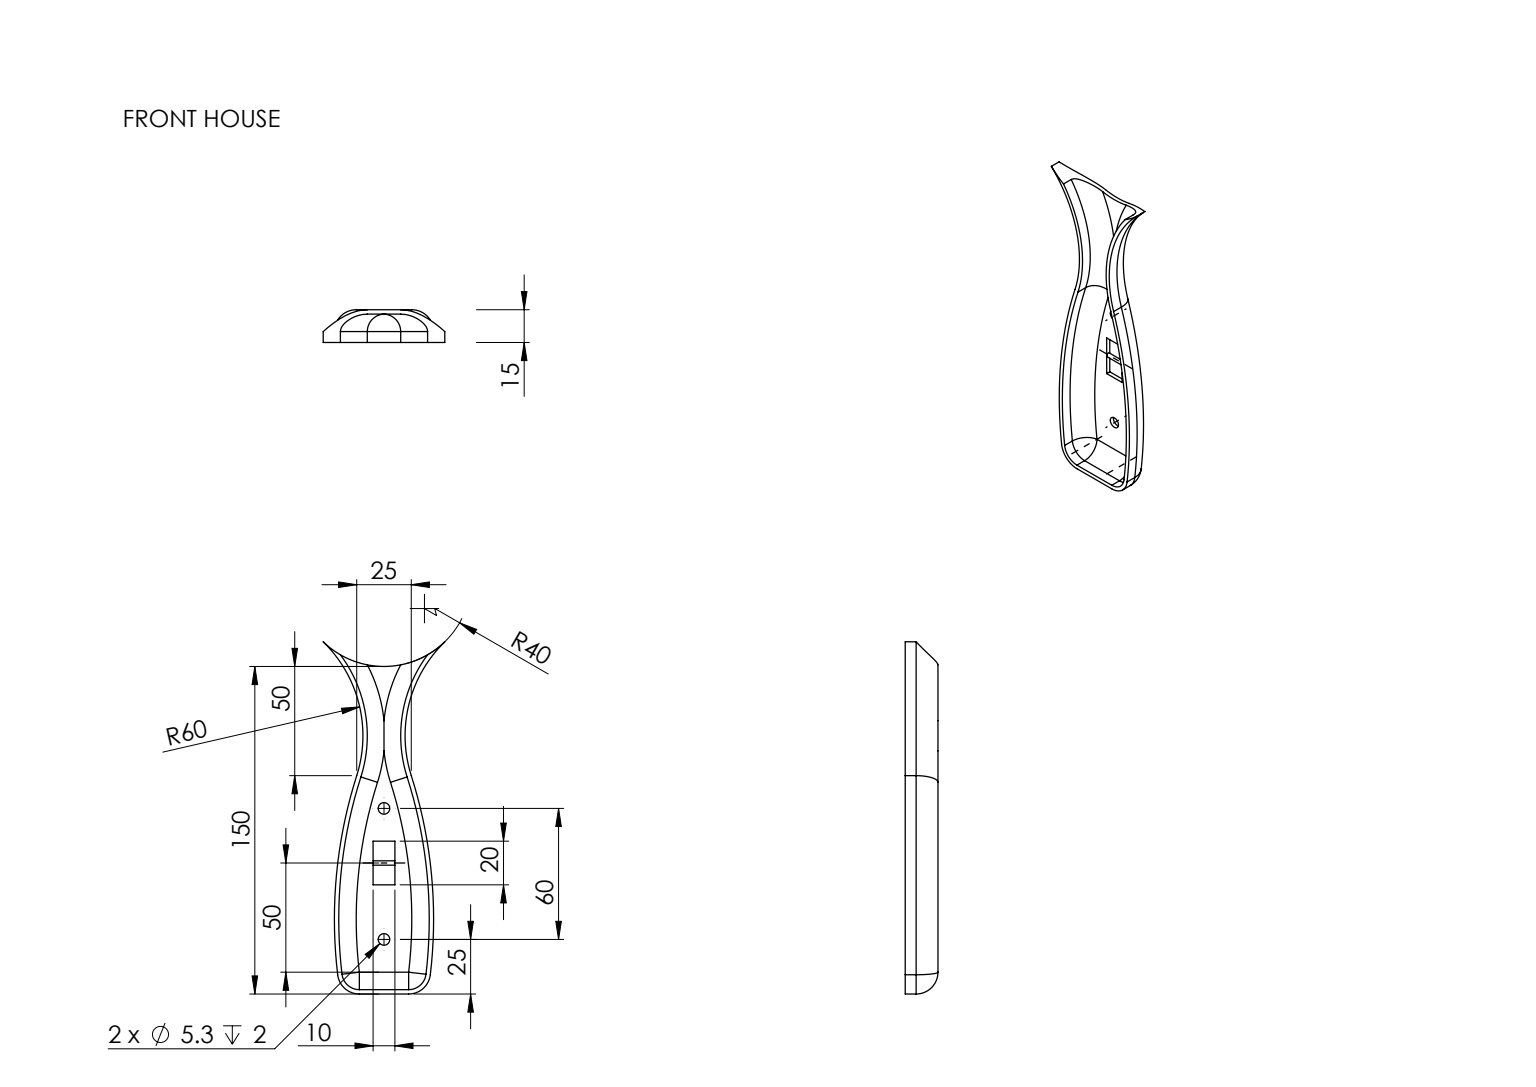
ISO-10303-21;
HEADER;
FILE_DESCRIPTION (('STEP AP214'),
    '1' );
FILE_NAME ('front house.step',
    '2026-10-04T13:31:42',
    ( '' ),
    ( '' ),
    'SwSTEP 2.0',
    'SolidWorks 2026',
    '' );
FILE_SCHEMA (( 'AUTOMOTIVE_DESIGN' ));
ENDSEC;

DATA;
#31=DIRECTION ( 'NONE',  ( 0.000000000000000000, 0.000000000000000000, 1.000000000000000000 ) ) ;
#221=EDGE_CURVE ( 'NONE', #165210, #193478, #178958, .T. ) ;
#227=CARTESIAN_POINT ( 'NONE',  ( 69.65682714487590488, -71.74905178543389184, -4.999999999999999112 ) ) ;
#394=ADVANCED_FACE ( 'NONE', ( #34064 ), #127044, .F. ) ;
#780=DIRECTION ( 'NONE',  ( 0.000000000000000000, 0.000000000000000000, 1.000000000000000000 ) ) ;
#955=EDGE_CURVE ( 'NONE', #12036, #40598, #167128, .T. ) ;
#999=ORIENTED_EDGE ( 'NONE', *, *, #31053, .F. ) ;
#1017=VECTOR ( 'NONE', #142739, 1000.000000000000000 ) ;
#1085=CARTESIAN_POINT ( 'NONE',  ( 2.973862142520697471, -93.04182470242777470, -4.999999999999999112 ) ) ;
#1208=CARTESIAN_POINT ( 'NONE',  ( -193.3062444957834884, -155.7167183371838064, -4.999999999999999112 ) ) ;
#1246=DIRECTION ( 'NONE',  ( 0.000000000000000000, 0.000000000000000000, -1.000000000000000000 ) ) ;
#1328=( LENGTH_UNIT ( ) NAMED_UNIT ( * ) SI_UNIT ( .MILLI., .METRE. ) );
#1396=AXIS2_PLACEMENT_3D ( 'NONE', #152271, #151292, #11796 ) ;
#1425=AXIS2_PLACEMENT_3D ( 'NONE', #179920, #53542, #83864 ) ;
#1725=ORIENTED_EDGE ( 'NONE', *, *, #84050, .T. ) ;
#1873=CARTESIAN_POINT ( 'NONE',  ( 18.50421606877890923, -35.46346162465770391, -8.316515678940758605 ) ) ;
#2039=ORIENTED_EDGE ( 'NONE', *, *, #94568, .T. ) ;
#2326=AXIS2_PLACEMENT_3D ( 'NONE', #102933, #86762, #132273 ) ;
#2374=CARTESIAN_POINT ( 'NONE',  ( 21.23184647844206197, -181.1785498424364675, 0.000000000000000000 ) ) ;
#2569=AXIS2_PLACEMENT_3D ( 'NONE', #195043, #118200, #101008 ) ;
#2600=CIRCLE ( 'NONE', #60618, 214.0437394197456342 ) ;
#3186=CARTESIAN_POINT ( 'NONE',  ( -4.999999999999999112, -140.0000000000000000, -15.00000000000000000 ) ) ;
#3248=FACE_OUTER_BOUND ( 'NONE', #133845, .T. ) ;
#3260=EDGE_CURVE ( 'NONE', #40834, #66675, #157727, .T. ) ;
#3607=CARTESIAN_POINT ( 'NONE',  ( 22.30855676328228654, -33.25042073255080766, -9.512168350472055778 ) ) ;
#3770=DIRECTION ( 'NONE',  ( 0.000000000000000000, 0.000000000000000000, 1.000000000000000000 ) ) ;
#3944=ORIENTED_EDGE ( 'NONE', *, *, #32795, .T. ) ;
#3998=DIRECTION ( 'NONE',  ( -0.1178549842436482503, 0.9930308165857338887, -1.226674847570000151E-16 ) ) ;
#4010=( NAMED_UNIT ( * ) SI_UNIT ( $, .STERADIAN. ) SOLID_ANGLE_UNIT ( ) );
#4197=DIRECTION ( 'NONE',  ( -1.000000000000000000, 0.000000000000000000, 0.000000000000000000 ) ) ;
#4394=EDGE_LOOP ( 'NONE', ( #77649, #111972, #192802, #188802 ) ) ;
#4402=ORIENTED_EDGE ( 'NONE', *, *, #164677, .T. ) ;
#4433=CARTESIAN_POINT ( 'NONE',  ( -4.622231866529366047E-30, -105.0000000000000000, -15.00000000000000000 ) ) ;
#4442=CARTESIAN_POINT ( 'NONE',  ( -7.652493125962417153, -39.26116846143397510, -13.00000000000000000 ) ) ;
#4543=CARTESIAN_POINT ( 'NONE',  ( -69.65682714487590488, -71.74905178543390605, -15.00000000000000000 ) ) ;
#4625=EDGE_CURVE ( 'NONE', #192038, #188447, #191917, .T. ) ;
#4663=CARTESIAN_POINT ( 'NONE',  ( -4.999999999999999112, -140.0000000000000000, -15.00000000000000000 ) ) ;
#4730=CIRCLE ( 'NONE', #36937, 214.0437394197456911 ) ;
#4808=ADVANCED_FACE ( 'NONE', ( #75423 ), #167452, .T. ) ;
#4872=ORIENTED_EDGE ( 'NONE', *, *, #119692, .T. ) ;
#5076=DIRECTION ( 'NONE',  ( 1.000000000000000000, -5.392603844284257652E-33, 0.000000000000000000 ) ) ;
#5235=CARTESIAN_POINT ( 'NONE',  ( 5.000000000000001776, -120.0000000000000142, 0.0009999999999992653654 ) ) ;
#5261=EDGE_CURVE ( 'NONE', #139926, #193517, #14400, .T. ) ;
#5267=FACE_OUTER_BOUND ( 'NONE', #180808, .T. ) ;
#5354=CIRCLE ( 'NONE', #118409, 40.00000000000002132 ) ;
#5434=CARTESIAN_POINT ( 'NONE',  ( -4.718528363748727840E-30, -105.0000000000000000, -13.00000000000000000 ) ) ;
#5444=CARTESIAN_POINT ( 'NONE',  ( -10.96632750431057879, -38.47313893329367573, -12.60384275245237617 ) ) ;
#5846=CARTESIAN_POINT ( 'NONE',  ( 14.06517603784871007, -37.45098900586879154, -11.50478690063030562 ) ) ;
#6002=( NAMED_UNIT ( * ) PLANE_ANGLE_UNIT ( ) SI_UNIT ( $, .RADIAN. ) );
#6237=DIRECTION ( 'NONE',  ( -5.392603844284257652E-33, 1.000000000000000000, 0.000000000000000000 ) ) ;
#6266=CYLINDRICAL_SURFACE ( 'NONE', #130179, 59.99999999999998579 ) ;
#6267=ORIENTED_EDGE ( 'NONE', *, *, #21840, .T. ) ;
#6497=DIRECTION ( 'NONE',  ( -1.000000000000000000, -4.336808689942018352E-17, 3.574525976782710619E-31 ) ) ;
#6556=DIRECTION ( 'NONE',  ( 0.000000000000000000, 0.000000000000000000, -1.000000000000000000 ) ) ;
#6627=VERTEX_POINT ( 'NONE', #57076 ) ;
#6820=FACE_OUTER_BOUND ( 'NONE', #145721, .T. ) ;
#6959=CARTESIAN_POINT ( 'NONE',  ( -9.720620470091368759, -38.81506340700470048, -14.89813575833734305 ) ) ;
#7058=MANIFOLD_SOLID_BREP ( 'AdvancedHole1', #101418 ) ;
#7224=DIRECTION ( 'NONE',  ( 1.000000000000000000, 0.000000000000000000, 0.000000000000000000 ) ) ;
#7386=EDGE_LOOP ( 'NONE', ( #176353, #78348, #99493, #52023, #74607 ) ) ;
#7454=LINE ( 'NONE', #67143, #166615 ) ;
#8020=DIRECTION ( 'NONE',  ( -1.000000000000000000, -5.267352820763006950E-15, 0.000000000000000000 ) ) ;
#8023=AXIS2_PLACEMENT_3D ( 'NONE', #149445, #135288, #120095 ) ;
#8299=ADVANCED_FACE ( 'NONE', ( #6820 ), #108199, .F. ) ;
#8310=EDGE_CURVE ( 'NONE', #132987, #99125, #22008, .T. ) ;
#8317=EDGE_LOOP ( 'NONE', ( #155924, #169926 ) ) ;
#8368=CIRCLE ( 'NONE', #104487, 69.99999999999997158 ) ;
#8438=ORIENTED_EDGE ( 'NONE', *, *, #48191, .F. ) ;
#8454=DIRECTION ( 'NONE',  ( -1.000000000000000000, 0.000000000000000000, 0.000000000000000000 ) ) ;
#8593=VERTEX_POINT ( 'NONE', #115010 ) ;
#8666=ORIENTED_EDGE ( 'NONE', *, *, #178067, .T. ) ;
#9000=CARTESIAN_POINT ( 'NONE',  ( -0.3431728551240714742, -71.74905178543389184, -4.999999999999999112 ) ) ;
#9041=CARTESIAN_POINT ( 'NONE',  ( 193.3062444957835453, -155.7167183371837496, -4.999999999999999112 ) ) ;
#9199=ADVANCED_FACE ( 'NONE', ( #12843 ), #74509, .F. ) ;
#9471=CARTESIAN_POINT ( 'NONE',  ( -18.05685959898565685, -35.69332804049738428, -8.787752958456431784 ) ) ;
#9484=DIRECTION ( 'NONE',  ( -1.000000000000000000, 4.336808689942018352E-17, 0.000000000000000000 ) ) ;
#9541=CARTESIAN_POINT ( 'NONE',  ( 5.000000000000000888, -140.0000000000000000, 0.0009999999999992653654 ) ) ;
#9567=DIRECTION ( 'NONE',  ( 0.000000000000000000, 0.000000000000000000, -1.000000000000000000 ) ) ;
#9619=CARTESIAN_POINT ( 'NONE',  ( 11.73776690369117937, -38.24261239843917082, -14.51832217641615586 ) ) ;
#9693=CARTESIAN_POINT ( 'NONE',  ( 19.97888994334924107, -34.65319547504297759, 0.000000000000000000 ) ) ;
#9945=PLANE ( 'NONE',  #95324 ) ;
#10213=CARTESIAN_POINT ( 'NONE',  ( -7.656827144875921753, -71.74905178543390605, -15.00000000000000000 ) ) ;
#10237=ORIENTED_EDGE ( 'NONE', *, *, #127999, .T. ) ;
#10262=FACE_OUTER_BOUND ( 'NONE', #193309, .T. ) ;
#10449=CARTESIAN_POINT ( 'NONE',  ( 5.000000000000000888, -140.0000000000000000, -15.00000000000000000 ) ) ;
#10474=ORIENTED_EDGE ( 'NONE', *, *, #142789, .T. ) ;
#10483=DIRECTION ( 'NONE',  ( 0.000000000000000000, -1.000000000000000000, 0.000000000000000000 ) ) ;
#10575=ADVANCED_FACE ( 'NONE', ( #143863 ), #188902, .T. ) ;
#10632=AXIS2_PLACEMENT_3D ( 'NONE', #1085, #62761, #79930 ) ;
#10770=CIRCLE ( 'NONE', #191582, 69.99999999999997158 ) ;
#11242=EDGE_LOOP ( 'NONE', ( #101594, #137434, #105999, #91375 ) ) ;
#11284=TOROIDAL_SURFACE ( 'NONE', #156599, 69.99999999999998579, 10.00000000000000000 ) ;
#11382=AXIS2_PLACEMENT_3D ( 'NONE', #132278, #86767, #89760 ) ;
#11477=CARTESIAN_POINT ( 'NONE',  ( -18.72120804366350555, -35.34920564451201841, -8.063943084929409366 ) ) ;
#11550=AXIS2_PLACEMENT_3D ( 'NONE', #60720, #15228, #76887 ) ;
#11796=DIRECTION ( 'NONE',  ( -1.000000000000000000, 5.392603844284257652E-33, 0.000000000000000000 ) ) ;
#11861=CARTESIAN_POINT ( 'NONE',  ( 5.000000000000000888, -140.0000000000000000, 0.0009999999999992653654 ) ) ;
#11911=CIRCLE ( 'NONE', #95864, 216.0437394197456911 ) ;
#11953=FACE_OUTER_BOUND ( 'NONE', #124538, .T. ) ;
#12010=PLANE ( 'NONE',  #96796 ) ;
#12035=CARTESIAN_POINT ( 'NONE',  ( 21.23184647844207618, -181.1785498424364675, -4.999999999999999112 ) ) ;
#12036=VERTEX_POINT ( 'NONE', #40450 ) ;
#12455=CIRCLE ( 'NONE', #177115, 216.0437394197456911 ) ;
#12473=CARTESIAN_POINT ( 'NONE',  ( -15.76296483128273707, -36.76812510865116934, -10.58138071059118701 ) ) ;
#12478=ORIENTED_EDGE ( 'NONE', *, *, #22446, .F. ) ;
#12843=FACE_OUTER_BOUND ( 'NONE', #7386, .T. ) ;
#12933=CARTESIAN_POINT ( 'NONE',  ( -3.573655867281984216E-15, 2.428612866367529932E-14, -13.00000000000000000 ) ) ;
#12963=DIRECTION ( 'NONE',  ( -1.000000000000000000, 0.000000000000000000, 0.000000000000000000 ) ) ;
#13167=ORIENTED_EDGE ( 'NONE', *, *, #59429, .F. ) ;
#13706=ADVANCED_FACE ( 'NONE', ( #135627 ), #151779, .T. ) ;
#13755=DIRECTION ( 'NONE',  ( -5.392603844284257652E-33, -1.000000000000000000, -0.000000000000000000 ) ) ;
#13813=ORIENTED_EDGE ( 'NONE', *, *, #31053, .T. ) ;
#13989=ORIENTED_EDGE ( 'NONE', *, *, #42025, .F. ) ;
#13996=EDGE_LOOP ( 'NONE', ( #152884, #135844, #78840, #26414, #124117, #87089 ) ) ;
#14043=ORIENTED_EDGE ( 'NONE', *, *, #118990, .F. ) ;
#14248=LINE ( 'NONE', #45591, #191110 ) ;
#14299=CARTESIAN_POINT ( 'NONE',  ( 5.000000000000001776, -130.0000000000000000, -15.00000000000000000 ) ) ;
#14379=ORIENTED_EDGE ( 'NONE', *, *, #143946, .T. ) ;
#14400=CIRCLE ( 'NONE', #49903, 1.000000000000000888 ) ;
#14416=FACE_OUTER_BOUND ( 'NONE', #72162, .T. ) ;
#14442=DIRECTION ( 'NONE',  ( 0.000000000000000000, 0.000000000000000000, 1.000000000000000000 ) ) ;
#14496=VERTEX_POINT ( 'NONE', #24871 ) ;
#14587=PRODUCT ( 'front house', 'front house', '', ( #99773 ) ) ;
#14624=EDGE_LOOP ( 'NONE', ( #60138, #151275, #103948, #169903 ) ) ;
#14670=ORIENTED_EDGE ( 'NONE', *, *, #30090, .T. ) ;
#15059=DIRECTION ( 'NONE',  ( -0.000000000000000000, -0.000000000000000000, 1.000000000000000000 ) ) ;
#15063=CARTESIAN_POINT ( 'NONE',  ( 19.97888994334922685, -34.65319547504297759, -5.000000000000000000 ) ) ;
#15156=ADVANCED_FACE ( 'NONE', ( #166377 ), #150081, .T. ) ;
#15228=DIRECTION ( 'NONE',  ( -1.000000000000000000, 4.336808689942018352E-17, 0.000000000000000000 ) ) ;
#15374=ORIENTED_EDGE ( 'NONE', *, *, #124070, .T. ) ;
#15380=VERTEX_POINT ( 'NONE', #151204 ) ;
#15470=EDGE_LOOP ( 'NONE', ( #127977, #132284 ) ) ;
#16009=CIRCLE ( 'NONE', #183867, 10.00000000000000000 ) ;
#16062=CARTESIAN_POINT ( 'NONE',  ( 18.71701949505375850, -35.35143465962271137, -8.069197253667519831 ) ) ;
#16115=AXIS2_PLACEMENT_3D ( 'NONE', #109939, #18939, #79600 ) ;
#16283=AXIS2_PLACEMENT_3D ( 'NONE', #142519, #3998, #65677 ) ;
#16324=CARTESIAN_POINT ( 'NONE',  ( 1.251854463851703304E-30, -64.82615989628266107, -13.00000000000000000 ) ) ;
#16357=DIRECTION ( 'NONE',  ( -0.000000000000000000, -0.000000000000000000, 1.000000000000000000 ) ) ;
#16373=ORIENTED_EDGE ( 'NONE', *, *, #128894, .T. ) ;
#16501=DIRECTION ( 'NONE',  ( -1.000000000000000000, -6.938893903907222461E-16, 0.000000000000000000 ) ) ;
#16889=LINE ( 'NONE', #110877, #51594 ) ;
#16962=CARTESIAN_POINT ( 'NONE',  ( -12.73749492396214578, -155.7167183371837496, -4.999999999999999112 ) ) ;
#17051=DIRECTION ( 'NONE',  ( 1.000000000000000000, -5.392603844284257652E-33, 0.000000000000000000 ) ) ;
#17054=FACE_BOUND ( 'NONE', #15470, .T. ) ;
#17119=CARTESIAN_POINT ( 'NONE',  ( 11.30153831258470731, -190.0000000000000000, -1.787262988391354872E-28 ) ) ;
#17206=DIRECTION ( 'NONE',  ( -1.084202172485503448E-15, 1.000000000000000000, 0.000000000000000000 ) ) ;
#17395=DIRECTION ( 'NONE',  ( -1.000000000000000000, 0.000000000000000000, 0.000000000000000000 ) ) ;
#17532=CARTESIAN_POINT ( 'NONE',  ( 69.65682714487590488, -71.74905178543389184, -15.00000000000000000 ) ) ;
#17665=CIRCLE ( 'NONE', #82280, 10.00000000000000000 ) ;
#17726=LINE ( 'NONE', #125887, #25441 ) ;
#17903=DIRECTION ( 'NONE',  ( 0.000000000000000000, 0.000000000000000000, 1.000000000000000000 ) ) ;
#17946=CIRCLE ( 'NONE', #134285, 216.0437394197456342 ) ;
#18248=DIRECTION ( 'NONE',  ( 0.000000000000000000, 0.000000000000000000, -1.000000000000000000 ) ) ;
#18328=ADVANCED_FACE ( 'NONE', ( #38549 ), #23381, .T. ) ;
#18602=ORIENTED_EDGE ( 'NONE', *, *, #70632, .T. ) ;
#18609=VECTOR ( 'NONE', #153495, 1000.000000000000000 ) ;
#18645=DIRECTION ( 'NONE',  ( -1.000000000000000000, 0.000000000000000000, 0.000000000000000000 ) ) ;
#18939=DIRECTION ( 'NONE',  ( 0.000000000000000000, 0.000000000000000000, -1.000000000000000000 ) ) ;
#19103=DIRECTION ( 'NONE',  ( 0.000000000000000000, 0.000000000000000000, -1.000000000000000000 ) ) ;
#19157=CARTESIAN_POINT ( 'NONE',  ( -2.649999999999999911, -165.0000000000000000, -13.00000000000000000 ) ) ;
#19169=CARTESIAN_POINT ( 'NONE',  ( -8.695239111463058279, -39.05792421784926916, -14.99999999999999822 ) ) ;
#19466=VERTEX_POINT ( 'NONE', #19157 ) ;
#19537=CARTESIAN_POINT ( 'NONE',  ( -193.3062444957834884, -155.7167183371838064, -4.999999999999999112 ) ) ;
#19615=DIRECTION ( 'NONE',  ( 1.000000000000000000, 0.000000000000000000, 0.000000000000000000 ) ) ;
#19643=UNCERTAINTY_MEASURE_WITH_UNIT (LENGTH_MEASURE( 1.000000000000000082E-05 ), #1328, 'distance_accuracy_value', 'NONE');
#19783=CARTESIAN_POINT ( 'NONE',  ( 13.21959898025320967, -37.75582843579748271, -14.12000380663810262 ) ) ;
#19836=VERTEX_POINT ( 'NONE', #130283 ) ;
#19856=CARTESIAN_POINT ( 'NONE',  ( 2.649999999999999911, -105.0000000000000000, -13.00000000000000000 ) ) ;
#19915=CARTESIAN_POINT ( 'NONE',  ( 5.000000000000000888, -131.0000000000000000, -13.99999999999999822 ) ) ;
#20029=CARTESIAN_POINT ( 'NONE',  ( 10.96715308212796458, -38.47291154382241274, -12.60366170504685712 ) ) ;
#20388=EDGE_LOOP ( 'NONE', ( #171344, #83609, #148692 ) ) ;
#20401=ORIENTED_EDGE ( 'NONE', *, *, #108955, .T. ) ;
#20623=CARTESIAN_POINT ( 'NONE',  ( -9.003469324749447722, -38.97944712463819883, -12.94545205561310119 ) ) ;
#20624=CIRCLE ( 'NONE', #91768, 8.000000000000000000 ) ;
#20723=LINE ( 'NONE', #144068, #186001 ) ;
#20852=AXIS2_PLACEMENT_3D ( 'NONE', #106884, #46212, #28098 ) ;
#21026=DIRECTION ( 'NONE',  ( -1.000000000000000000, 0.000000000000000000, 0.000000000000000000 ) ) ;
#21060=ORIENTED_EDGE ( 'NONE', *, *, #135206, .T. ) ;
#21105=CARTESIAN_POINT ( 'NONE',  ( 11.30153831258469843, -180.0000000000000000, -4.999999999999999112 ) ) ;
#21171=CIRCLE ( 'NONE', #11550, 1.000000000000000888 ) ;
#21682=CIRCLE ( 'NONE', #192727, 1.000000000000000888 ) ;
#21713=ORIENTED_EDGE ( 'NONE', *, *, #40967, .F. ) ;
#21840=EDGE_CURVE ( 'NONE', #125859, #167341, #21171, .T. ) ;
#21881=ORIENTED_EDGE ( 'NONE', *, *, #82288, .T. ) ;
#22008=LINE ( 'NONE', #162510, #85543 ) ;
#22026=CARTESIAN_POINT ( 'NONE',  ( 9.003517414636718286, -38.97943997941770533, -12.94545749024833547 ) ) ;
#22118=CARTESIAN_POINT ( 'NONE',  ( 11.30153831258470731, -188.0000000000000000, -4.999999999999999112 ) ) ;
#22345=ORIENTED_EDGE ( 'NONE', *, *, #44596, .F. ) ;
#22381=CARTESIAN_POINT ( 'NONE',  ( -69.65682714487590488, -71.74905178543390605, -15.00000000000000000 ) ) ;
#22446=EDGE_CURVE ( 'NONE', #197949, #150223, #139302, .T. ) ;
#22488=AXIS2_PLACEMENT_3D ( 'NONE', #169792, #19103, #171788 ) ;
#22637=VERTEX_POINT ( 'NONE', #30144 ) ;
#22697=ORIENTED_EDGE ( 'NONE', *, *, #25125, .T. ) ;
#22869=ORIENTED_EDGE ( 'NONE', *, *, #178067, .F. ) ;
#23028=CARTESIAN_POINT ( 'NONE',  ( 10.31991442469048614, -38.65177141104609149, -12.74737010625873523 ) ) ;
#23117=VERTEX_POINT ( 'NONE', #198529 ) ;
#23152=CARTESIAN_POINT ( 'NONE',  ( -26.21509334545639192, -30.21538139615938334, -6.441305576064758398 ) ) ;
#23189=( NAMED_UNIT ( * ) SI_UNIT ( $, .STERADIAN. ) SOLID_ANGLE_UNIT ( ) );
#23191=EDGE_LOOP ( 'NONE', ( #102945, #168389, #1725, #52952, #125256 ) ) ;
#23213=CARTESIAN_POINT ( 'NONE',  ( -11.30153831258471975, -180.0000000000000000, -4.999999999999999112 ) ) ;
#23381=CYLINDRICAL_SURFACE ( 'NONE', #59719, 61.99999999999998579 ) ;
#23400=ORIENTED_EDGE ( 'NONE', *, *, #157314, .T. ) ;
#23533=DIRECTION ( 'NONE',  ( 0.000000000000000000, 0.000000000000000000, 1.000000000000000000 ) ) ;
#23638=ORIENTED_EDGE ( 'NONE', *, *, #148455, .T. ) ;
#23668=DIRECTION ( 'NONE',  ( 0.000000000000000000, 0.000000000000000000, -1.000000000000000000 ) ) ;
#23790=EDGE_CURVE ( 'NONE', #122541, #40748, #25901, .T. ) ;
#23850=DIRECTION ( 'NONE',  ( -1.000000000000000000, 0.000000000000000000, 0.000000000000000000 ) ) ;
#23912=ORIENTED_EDGE ( 'NONE', *, *, #106542, .F. ) ;
#23972=CIRCLE ( 'NONE', #30321, 206.0437394197456911 ) ;
#24026=CARTESIAN_POINT ( 'NONE',  ( -6.856101608890825108E-16, -71.74905178543389184, -12.99263613531267936 ) ) ;
#24352=ORIENTED_EDGE ( 'NONE', *, *, #42529, .T. ) ;
#24717=DIRECTION ( 'NONE',  ( 4.336808689942017120E-17, 1.000000000000000000, 0.000000000000000000 ) ) ;
#24871=CARTESIAN_POINT ( 'NONE',  ( 2.649999999999999911, -165.0000000000000000, -13.00000000000000000 ) ) ;
#24925=ORIENTED_EDGE ( 'NONE', *, *, #54327, .F. ) ;
#25021=ORIENTED_EDGE ( 'NONE', *, *, #3260, .T. ) ;
#25032=AXIS2_PLACEMENT_3D ( 'NONE', #79551, #186762, #171571 ) ;
#25084=EDGE_CURVE ( 'NONE', #182160, #27470, #78080, .T. ) ;
#25125=EDGE_CURVE ( 'NONE', #125859, #133361, #62915, .T. ) ;
#25148=FACE_OUTER_BOUND ( 'NONE', #147177, .T. ) ;
#25149=CARTESIAN_POINT ( 'NONE',  ( 5.000000000000001776, -120.0000000000000142, -15.00000000000000000 ) ) ;
#25157=EDGE_LOOP ( 'NONE', ( #86325, #134189, #138051, #172711, #183482 ) ) ;
#25181=CARTESIAN_POINT ( 'NONE',  ( -3.573655867281984216E-15, 2.428612866367529932E-14, -13.00000000000000000 ) ) ;
#25330=ADVANCED_FACE ( 'NONE', ( #5267 ), #6266, .F. ) ;
#25441=VECTOR ( 'NONE', #187587, 1000.000000000000000 ) ;
#25798=CARTESIAN_POINT ( 'NONE',  ( 9.720660689315817393, -38.81505388558687031, -14.89813180556192407 ) ) ;
#25821=CIRCLE ( 'NONE', #190601, 2.649999999999999911 ) ;
#25901=LINE ( 'NONE', #180586, #110722 ) ;
#26124=ORIENTED_EDGE ( 'NONE', *, *, #154768, .T. ) ;
#26379=ORIENTED_EDGE ( 'NONE', *, *, #82917, .F. ) ;
#26414=ORIENTED_EDGE ( 'NONE', *, *, #118990, .T. ) ;
#26478=DIRECTION ( 'NONE',  ( -0.000000000000000000, -0.000000000000000000, 1.000000000000000000 ) ) ;
#26668=ADVANCED_FACE ( 'NONE', ( #32411 ), #94248, .T. ) ;
#26924=ORIENTED_EDGE ( 'NONE', *, *, #107568, .F. ) ;
#27145=CARTESIAN_POINT ( 'NONE',  ( -193.3062444957834884, -155.7167183371838064, -13.00000000000000000 ) ) ;
#27198=ORIENTED_EDGE ( 'NONE', *, *, #43624, .T. ) ;
#27389=LINE ( 'NONE', #181073, #94965 ) ;
#27433=EDGE_CURVE ( 'NONE', #96037, #182127, #14248, .T. ) ;
#27470=VERTEX_POINT ( 'NONE', #137595 ) ;
#27838=VERTEX_POINT ( 'NONE', #54551 ) ;
#28098=DIRECTION ( 'NONE',  ( -1.000000000000000000, 0.000000000000000000, 0.000000000000000000 ) ) ;
#28184=TOROIDAL_SURFACE ( 'NONE', #53977, 69.99999999999998579, 10.00000000000000000 ) ;
#28296=DIRECTION ( 'NONE',  ( -1.000000000000000000, 0.000000000000000000, 5.421010862427522170E-16 ) ) ;
#28369=AXIS2_PLACEMENT_3D ( 'NONE', #56430, #118110, #135280 ) ;
#28497=ORIENTED_EDGE ( 'NONE', *, *, #128725, .F. ) ;
#28587=ORIENTED_EDGE ( 'NONE', *, *, #116598, .T. ) ;
#28615=CIRCLE ( 'NONE', #73781, 1.000000000000000888 ) ;
#28634=CARTESIAN_POINT ( 'NONE',  ( -17.82155712959115590, -35.81153309740783897, -9.011975243048143014 ) ) ;
#28640=ORIENTED_EDGE ( 'NONE', *, *, #42025, .T. ) ;
#28648=DIRECTION ( 'NONE',  ( 1.000000000000000000, 0.000000000000000000, 0.000000000000000000 ) ) ;
#29111=CARTESIAN_POINT ( 'NONE',  ( -69.65682714487590488, -71.74905178543390605, -13.00000000000000000 ) ) ;
#29170=DIRECTION ( 'NONE',  ( -1.000000000000000000, -4.336808689942018352E-17, 3.574525976782710181E-31 ) ) ;
#29199=DIRECTION ( 'NONE',  ( 0.000000000000000000, 0.000000000000000000, -1.000000000000000000 ) ) ;
#29337=DIRECTION ( 'NONE',  ( -1.000000000000000000, 0.000000000000000000, 5.421010862427522170E-16 ) ) ;
#29479=FACE_OUTER_BOUND ( 'NONE', #30544, .T. ) ;
#29607=CARTESIAN_POINT ( 'NONE',  ( -19.91688362670921464, -34.68888220807522060, -5.694635852519195574 ) ) ;
#29727=DIRECTION ( 'NONE',  ( -1.000000000000000000, -1.249000902703301424E-14, 0.000000000000000000 ) ) ;
#29958=AXIS2_PLACEMENT_3D ( 'NONE', #118743, #9567, #194585 ) ;
#30088=VERTEX_POINT ( 'NONE', #48825 ) ;
#30090=EDGE_CURVE ( 'NONE', #164159, #164433, #169494, .T. ) ;
#30144=CARTESIAN_POINT ( 'NONE',  ( -7.656827144875921753, -71.74905178543390605, 8.936314941956774358E-29 ) ) ;
#30281=ADVANCED_FACE ( 'NONE', ( #76922 ), #45603, .T. ) ;
#30321=AXIS2_PLACEMENT_3D ( 'NONE', #83033, #51708, #157903 ) ;
#30544=EDGE_LOOP ( 'NONE', ( #24925, #25021, #101661, #82248 ) ) ;
#30615=CARTESIAN_POINT ( 'NONE',  ( -4.622231866529366047E-30, -105.0000000000000000, -15.00000000000000000 ) ) ;
#30626=DIRECTION ( 'NONE',  ( -0.3041824702427683436, -0.9526137857479322069, 2.960637879548173518E-15 ) ) ;
#30881=ORIENTED_EDGE ( 'NONE', *, *, #48487, .T. ) ;
#31053=EDGE_CURVE ( 'NONE', #182127, #147958, #17665, .T. ) ;
#31395=CARTESIAN_POINT ( 'NONE',  ( 12.50000000000001066, -90.00000000000005684, -15.00000000000000000 ) ) ;
#31538=ORIENTED_EDGE ( 'NONE', *, *, #128894, .F. ) ;
#31597=ORIENTED_EDGE ( 'NONE', *, *, #23790, .F. ) ;
#31615=VECTOR ( 'NONE', #95742, 1000.000000000000000 ) ;
#31652=ORIENTED_EDGE ( 'NONE', *, *, #83840, .F. ) ;
#31658=ORIENTED_EDGE ( 'NONE', *, *, #4625, .T. ) ;
#31768=AXIS2_PLACEMENT_3D ( 'NONE', #16962, #78615, #140290 ) ;
#31782=LINE ( 'NONE', #90464, #172810 ) ;
#32170=CIRCLE ( 'NONE', #64493, 10.00000000000000178 ) ;
#32224=FACE_OUTER_BOUND ( 'NONE', #179278, .T. ) ;
#32359=LINE ( 'NONE', #138529, #51628 ) ;
#32389=EDGE_LOOP ( 'NONE', ( #162936, #185817, #77336, #138820, #96284, #163282, #32536, #177807, #21713, #188073, #165154, #129216, #80845, #178640, #143786, #2039, #107041, #13813, #23638, #96495 ) ) ;
#32411=FACE_OUTER_BOUND ( 'NONE', #25157, .T. ) ;
#32446=DIRECTION ( 'NONE',  ( -1.000000000000000000, 1.154084784954514691E-14, 0.000000000000000000 ) ) ;
#32518=CARTESIAN_POINT ( 'NONE',  ( 5.035744501201078851E-13, -76.33743099897125717, -12.99988689144064402 ) ) ;
#32536=ORIENTED_EDGE ( 'NONE', *, *, #25084, .F. ) ;
#32795=EDGE_CURVE ( 'NONE', #41468, #92045, #152540, .T. ) ;
#32804=FACE_OUTER_BOUND ( 'NONE', #112589, .T. ) ;
#33042=CARTESIAN_POINT ( 'NONE',  ( 69.65682714487590488, -71.74905178543389184, -4.999999999999999112 ) ) ;
#33072=VERTEX_POINT ( 'NONE', #199051 ) ;
#33538=DIRECTION ( 'NONE',  ( -1.000000000000000000, -4.336808689942018352E-17, 3.574525976782710619E-31 ) ) ;
#33882=( GEOMETRIC_REPRESENTATION_CONTEXT ( 3 ) GLOBAL_UNCERTAINTY_ASSIGNED_CONTEXT ( ( #19643 ) ) GLOBAL_UNIT_ASSIGNED_CONTEXT ( ( #1328, #108521, #121702 ) ) REPRESENTATION_CONTEXT ( 'NONE', 'WORKASPACE' ) );
#33887=CARTESIAN_POINT ( 'NONE',  ( 11.30153831258469843, -180.0000000000000000, -13.00000000000000000 ) ) ;
#33912=AXIS2_PLACEMENT_3D ( 'NONE', #137756, #62894, #167124 ) ;
#34058=DIRECTION ( 'NONE',  ( 1.000000000000000000, 0.000000000000000000, 0.000000000000000000 ) ) ;
#34064=FACE_OUTER_BOUND ( 'NONE', #131281, .T. ) ;
#34145=EDGE_LOOP ( 'NONE', ( #113933, #104667, #129575, #111356 ) ) ;
#34170=EDGE_CURVE ( 'NONE', #182160, #171657, #149107, .T. ) ;
#34219=B_SPLINE_CURVE_WITH_KNOTS ( 'NONE', 3,
 ( #140219, #60398, #124049, #139232, #44255, #106902, #125065 ),
 .UNSPECIFIED., .F., .F.,
 ( 4, 3, 4 ),
 ( -4.508036450095025827E-05, 0.000000000000000000, 0.006877813788783073562 ),
 .UNSPECIFIED. ) ;
#34302=ORIENTED_EDGE ( 'NONE', *, *, #62612, .F. ) ;
#34395=DIRECTION ( 'NONE',  ( 0.000000000000000000, 0.000000000000000000, -1.000000000000000000 ) ) ;
#34532=AXIS2_PLACEMENT_3D ( 'NONE', #151543, #29199, #150553 ) ;
#34751=CARTESIAN_POINT ( 'NONE',  ( 5.000000000000000888, -140.0000000000000000, -15.00000000000000000 ) ) ;
#34859=LINE ( 'NONE', #158204, #66850 ) ;
#34953=CARTESIAN_POINT ( 'NONE',  ( 15.58367361853946065, -36.85270801516746531, -13.27795824800661961 ) ) ;
#35065=DIRECTION ( 'NONE',  ( 0.000000000000000000, -1.000000000000000000, 0.000000000000000000 ) ) ;
#35254=DIRECTION ( 'NONE',  ( 0.000000000000000000, 0.000000000000000000, -1.000000000000000000 ) ) ;
#35320=CARTESIAN_POINT ( 'NONE',  ( -7.652493125987827050, -39.26116846142902261, -15.00000000000000000 ) ) ;
#35850=DIRECTION ( 'NONE',  ( 4.336808689942018352E-17, -1.000000000000000000, 0.000000000000000000 ) ) ;
#36160=ORIENTED_EDGE ( 'NONE', *, *, #23790, .T. ) ;
#36346=VERTEX_POINT ( 'NONE', #193366 ) ;
#36494=ORIENTED_EDGE ( 'NONE', *, *, #163970, .F. ) ;
#36756=CARTESIAN_POINT ( 'NONE',  ( -11.30153831258470731, -180.0000000000000000, -15.00000000000000000 ) ) ;
#36931=CARTESIAN_POINT ( 'NONE',  ( 27.21324236920355233, -29.31705316289551533, -5.578213269879590541 ) ) ;
#36937=AXIS2_PLACEMENT_3D ( 'NONE', #38383, #70723, #132390 ) ;
#36969=ORIENTED_EDGE ( 'NONE', *, *, #58065, .F. ) ;
#37089=CARTESIAN_POINT ( 'NONE',  ( 11.30153831258470731, -180.0000000000000000, -15.00000000000000000 ) ) ;
#37267=DIRECTION ( 'NONE',  ( 0.9930308165857338887, -0.1178549842436482226, 0.000000000000000000 ) ) ;
#37365=AXIS2_PLACEMENT_3D ( 'NONE', #33042, #173550, #125047 ) ;
#37428=DIRECTION ( 'NONE',  ( 0.000000000000000000, 0.000000000000000000, -1.000000000000000000 ) ) ;
#37611=DIRECTION ( 'NONE',  ( 0.000000000000000000, 0.000000000000000000, 1.000000000000000000 ) ) ;
#37781=DIRECTION ( 'NONE',  ( 0.000000000000000000, 0.000000000000000000, -1.000000000000000000 ) ) ;
#37820=CARTESIAN_POINT ( 'NONE',  ( 69.65682714487590488, -71.74905178543389184, -4.999999999999999112 ) ) ;
#38038=VERTEX_POINT ( 'NONE', #172430 ) ;
#38095=DIRECTION ( 'NONE',  ( 0.000000000000000000, -1.000000000000000000, 0.000000000000000000 ) ) ;
#38347=EDGE_CURVE ( 'NONE', #158522, #164433, #63253, .T. ) ;
#38383=CARTESIAN_POINT ( 'NONE',  ( 193.3062444957835453, -155.7167183371837496, -4.999999999999999112 ) ) ;
#38544=DIRECTION ( 'NONE',  ( 5.392603844284257652E-33, -1.000000000000000000, 0.000000000000000000 ) ) ;
#38549=FACE_OUTER_BOUND ( 'NONE', #157737, .T. ) ;
#38658=ORIENTED_EDGE ( 'NONE', *, *, #8310, .F. ) ;
#38779=CYLINDRICAL_SURFACE ( 'NONE', #114874, 10.00000000000000000 ) ;
#38864=VERTEX_POINT ( 'NONE', #97541 ) ;
#38962=EDGE_CURVE ( 'NONE', #197193, #8593, #20723, .T. ) ;
#39019=DIRECTION ( 'NONE',  ( -1.000000000000000000, 0.000000000000000000, 0.000000000000000000 ) ) ;
#39055=DIRECTION ( 'NONE',  ( 0.000000000000000000, 1.000000000000000000, 0.000000000000000000 ) ) ;
#39085=DIRECTION ( 'NONE',  ( 1.000000000000000000, 0.000000000000000000, 0.000000000000000000 ) ) ;
#39169=CARTESIAN_POINT ( 'NONE',  ( -193.3062444957834884, -155.7167183371838064, -4.999999999999999112 ) ) ;
#39241=CARTESIAN_POINT ( 'NONE',  ( 2.973862142520690366, -93.04182470242774627, -15.00000000000000000 ) ) ;
#39357=EDGE_CURVE ( 'NONE', #64290, #97924, #63303, .T. ) ;
#39462=CARTESIAN_POINT ( 'NONE',  ( 10.59477242850415024, -90.60836494048558620, -15.00000000000000000 ) ) ;
#39488=DIRECTION ( 'NONE',  ( 0.000000000000000000, 0.000000000000000000, -1.000000000000000000 ) ) ;
#40245=DIRECTION ( 'NONE',  ( 0.000000000000000000, 0.000000000000000000, 1.000000000000000000 ) ) ;
#40292=LINE ( 'NONE', #25149, #179287 ) ;
#40357=VERTEX_POINT ( 'NONE', #68108 ) ;
#40450=CARTESIAN_POINT ( 'NONE',  ( -5.000000000000000000, -120.0000000000000142, -13.00000000000000000 ) ) ;
#40543=LINE ( 'NONE', #10213, #131638 ) ;
#40598=VERTEX_POINT ( 'NONE', #98428 ) ;
#40687=CARTESIAN_POINT ( 'NONE',  ( 1.348150961071065097E-30, -64.82615989628266107, -15.00000000000000000 ) ) ;
#40697=CARTESIAN_POINT ( 'NONE',  ( -193.3062444957834884, -155.7167183371838064, 0.000000000000000000 ) ) ;
#40705=AXIS2_PLACEMENT_3D ( 'NONE', #120589, #182284, #105428 ) ;
#40748=VERTEX_POINT ( 'NONE', #4663 ) ;
#40834=VERTEX_POINT ( 'NONE', #19856 ) ;
#40947=DIRECTION ( 'NONE',  ( 0.000000000000000000, 0.000000000000000000, -1.000000000000000000 ) ) ;
#40967=EDGE_CURVE ( 'NONE', #19836, #70507, #117665, .T. ) ;
#41329=CARTESIAN_POINT ( 'NONE',  ( -3.573655867282028392E-15, 2.428612866367529932E-14, 1.984260520772446048E-44 ) ) ;
#41393=CARTESIAN_POINT ( 'NONE',  ( -6.856101608890819192E-16, -64.85304063214812231, -12.99999966871702917 ) ) ;
#41468=VERTEX_POINT ( 'NONE', #9693 ) ;
#41630=VERTEX_POINT ( 'NONE', #122815 ) ;
#41803=CARTESIAN_POINT ( 'NONE',  ( -14.64368186514533932, -37.22806287882965393, -11.21878843496574518 ) ) ;
#41850=CARTESIAN_POINT ( 'NONE',  ( -10.59477242850411649, -90.60836494048552936, -15.00000000000000000 ) ) ;
#42025=EDGE_CURVE ( 'NONE', #23117, #188447, #67991, .T. ) ;
#42318=CARTESIAN_POINT ( 'NONE',  ( -69.65682714487590488, -71.74905178543390605, -15.00000000000000000 ) ) ;
#42529=EDGE_CURVE ( 'NONE', #15380, #38864, #93839, .T. ) ;
#42806=ORIENTED_EDGE ( 'NONE', *, *, #178304, .T. ) ;
#42893=CYLINDRICAL_SURFACE ( 'NONE', #29958, 2.649999999999999911 ) ;
#42899=FILL_AREA_STYLE_COLOUR ( '', #143549 ) ;
#42917=VECTOR ( 'NONE', #780, 1000.000000000000000 ) ;
#43273=ORIENTED_EDGE ( 'NONE', *, *, #128725, .T. ) ;
#43478=EDGE_CURVE ( 'NONE', #164159, #132746, #23972, .T. ) ;
#43624=EDGE_CURVE ( 'NONE', #164433, #133568, #59459, .T. ) ;
#43693=AXIS2_PLACEMENT_3D ( 'NONE', #156399, #17903, #34058 ) ;
#43764=FACE_OUTER_BOUND ( 'NONE', #83531, .T. ) ;
#43775=CARTESIAN_POINT ( 'NONE',  ( -19.99999999999998224, -188.0000000000000000, -15.00000000000000000 ) ) ;
#43824=VERTEX_POINT ( 'NONE', #80056 ) ;
#43910=DIRECTION ( 'NONE',  ( 0.000000000000000000, 0.000000000000000000, -1.000000000000000000 ) ) ;
#43996=EDGE_CURVE ( 'NONE', #65708, #70507, #27389, .T. ) ;
#44030=AXIS2_PLACEMENT_3D ( 'NONE', #121322, #90966, #29337 ) ;
#44066=ORIENTED_EDGE ( 'NONE', *, *, #143733, .T. ) ;
#44072=TOROIDAL_SURFACE ( 'NONE', #79554, 206.0437394197456911, 8.000000000000000000 ) ;
#44255=CARTESIAN_POINT ( 'NONE',  ( -1.114781414664558017E-12, -67.16384485484803690, -14.99989890117360503 ) ) ;
#44325=DIRECTION ( 'NONE',  ( -0.000000000000000000, -0.000000000000000000, 1.000000000000000000 ) ) ;
#44359=CIRCLE ( 'NONE', #109002, 69.99999999999998579 ) ;
#44370=DIRECTION ( 'NONE',  ( 0.000000000000000000, 0.000000000000000000, -1.000000000000000000 ) ) ;
#44569=DIRECTION ( 'NONE',  ( 0.000000000000000000, 0.000000000000000000, -1.000000000000000000 ) ) ;
#44596=EDGE_CURVE ( 'NONE', #151167, #36346, #51363, .T. ) ;
#44756=AXIS2_PLACEMENT_3D ( 'NONE', #129087, #112934, #191777 ) ;
#44969=ORIENTED_EDGE ( 'NONE', *, *, #148455, .F. ) ;
#45274=AXIS2_PLACEMENT_3D ( 'NONE', #53186, #101690, #129015 ) ;
#45527=CYLINDRICAL_SURFACE ( 'NONE', #46454, 40.00000000000002132 ) ;
#45591=CARTESIAN_POINT ( 'NONE',  ( 11.30153831258470731, -190.0000000000000000, -15.00000000000000000 ) ) ;
#45603=CYLINDRICAL_SURFACE ( 'NONE', #195359, 1.000000000000000888 ) ;
#45744=DIRECTION ( 'NONE',  ( 1.000000000000000000, 0.000000000000000000, 0.000000000000000000 ) ) ;
#45839=CARTESIAN_POINT ( 'NONE',  ( -2.649999999999999911, -105.0000000000000000, -15.00000000000000000 ) ) ;
#46184=ORIENTED_EDGE ( 'NONE', *, *, #97135, .F. ) ;
#46212=DIRECTION ( 'NONE',  ( 0.000000000000000000, 0.000000000000000000, -1.000000000000000000 ) ) ;
#46297=ORIENTED_EDGE ( 'NONE', *, *, #73681, .F. ) ;
#46454=AXIS2_PLACEMENT_3D ( 'NONE', #107181, #168852, #21026 ) ;
#46506=EDGE_CURVE ( 'NONE', #74166, #101229, #117487, .T. ) ;
#46614=CIRCLE ( 'NONE', #120942, 59.99999999999998579 ) ;
#46706=AXIS2_PLACEMENT_3D ( 'NONE', #134024, #193705, #23850 ) ;
#46742=MECHANICAL_DESIGN_GEOMETRIC_PRESENTATION_REPRESENTATION('',(#91879),#53220);
#46776=FACE_OUTER_BOUND ( 'NONE', #71687, .T. ) ;
#46835=PLANE ( 'NONE',  #153741 ) ;
#47004=AXIS2_PLACEMENT_3D ( 'NONE', #175896, #34395, #67705 ) ;
#47239=AXIS2_PLACEMENT_3D ( 'NONE', #101463, #9484, #10483 ) ;
#47328=ORIENTED_EDGE ( 'NONE', *, *, #168827, .F. ) ;
#47384=EDGE_LOOP ( 'NONE', ( #170476, #79382, #115140, #179154, #163179 ) ) ;
#47587=CARTESIAN_POINT ( 'NONE',  ( 69.65682714487590488, -71.74905178543389184, -4.999999999999999112 ) ) ;
#47791=DIRECTION ( 'NONE',  ( 0.9526137857479322069, -0.3041824702427683991, 0.000000000000000000 ) ) ;
#47812=EDGE_CURVE ( 'NONE', #41630, #40834, #165999, .T. ) ;
#47948=ORIENTED_EDGE ( 'NONE', *, *, #58065, .T. ) ;
#48103=DIRECTION ( 'NONE',  ( -1.000000000000000000, -4.336808689942018352E-17, 3.574525976782710619E-31 ) ) ;
#48165=AXIS2_PLACEMENT_3D ( 'NONE', #67764, #37428, #175959 ) ;
#48191=EDGE_CURVE ( 'NONE', #23117, #171657, #120801, .T. ) ;
#48243=EDGE_CURVE ( 'NONE', #165210, #188443, #20624, .T. ) ;
#48396=CARTESIAN_POINT ( 'NONE',  ( 16.30563709075146761, -36.53016886171239719, -10.22897874253568773 ) ) ;
#48487=EDGE_CURVE ( 'NONE', #122541, #169284, #174867, .T. ) ;
#48735=CARTESIAN_POINT ( 'NONE',  ( 10.59477242850415024, -90.60836494048558620, -4.999999999999999112 ) ) ;
#48825=CARTESIAN_POINT ( 'NONE',  ( 12.50000000000001066, -90.00000000000005684, 0.000000000000000000 ) ) ;
#49138=CARTESIAN_POINT ( 'NONE',  ( 27.86273085795036408, -28.69962071417356242, -4.999999999999999112 ) ) ;
#49277=DIRECTION ( 'NONE',  ( 0.9930308165857338887, 0.1178549842436489581, 0.000000000000000000 ) ) ;
#49280=CARTESIAN_POINT ( 'NONE',  ( 20.73749492396215288, -155.7167183371838064, -4.999999999999999112 ) ) ;
#49356=ORIENTED_EDGE ( 'NONE', *, *, #25125, .F. ) ;
#49543=DIRECTION ( 'NONE',  ( 0.000000000000000000, 0.000000000000000000, 1.000000000000000000 ) ) ;
#49544=ORIENTED_EDGE ( 'NONE', *, *, #166153, .T. ) ;
#49746=CARTESIAN_POINT ( 'NONE',  ( 5.000000000000000888, -140.0000000000000000, -13.00000000000000000 ) ) ;
#49756=VERTEX_POINT ( 'NONE', #167678 ) ;
#49903=AXIS2_PLACEMENT_3D ( 'NONE', #154283, #48103, #109759 ) ;
#50057=( GEOMETRIC_REPRESENTATION_CONTEXT ( 3 ) GLOBAL_UNCERTAINTY_ASSIGNED_CONTEXT ( ( #159130 ) ) GLOBAL_UNIT_ASSIGNED_CONTEXT ( ( #82837, #6002, #23189 ) ) REPRESENTATION_CONTEXT ( 'NONE', 'WORKASPACE' ) );
#50192=EDGE_CURVE ( 'NONE', #57973, #60209, #149973, .T. ) ;
#50279=CARTESIAN_POINT ( 'NONE',  ( 193.3062444957835453, -155.7167183371837496, -4.999999999999999112 ) ) ;
#50678=EDGE_CURVE ( 'NONE', #41630, #151273, #130085, .T. ) ;
#50976=EDGE_CURVE ( 'NONE', #30088, #36346, #46614, .T. ) ;
#50985=CARTESIAN_POINT ( 'NONE',  ( 69.65682714487590488, -71.74905178543389184, -4.999999999999999112 ) ) ;
#51152=ORIENTED_EDGE ( 'NONE', *, *, #143946, .F. ) ;
#51200=DIRECTION ( 'NONE',  ( 0.000000000000000000, 0.000000000000000000, -1.000000000000000000 ) ) ;
#51280=CARTESIAN_POINT ( 'NONE',  ( -2.649999999999999911, -105.0000000000000000, -15.00000000000000000 ) ) ;
#51322=DIRECTION ( 'NONE',  ( 1.908195823574487804E-15, 0.000000000000000000, -1.000000000000000000 ) ) ;
#51327=AXIS2_PLACEMENT_3D ( 'NONE', #1208, #184262, #45744 ) ;
#51363=LINE ( 'NONE', #160535, #198310 ) ;
#51484=CARTESIAN_POINT ( 'NONE',  ( -20.76432162245589907, -34.24133103601445072, -10.56798276756222599 ) ) ;
#51594=VECTOR ( 'NONE', #82511, 1000.000000000000000 ) ;
#51628=VECTOR ( 'NONE', #110184, 1000.000000000000000 ) ;
#51708=DIRECTION ( 'NONE',  ( 0.000000000000000000, 0.000000000000000000, -1.000000000000000000 ) ) ;
#51756=ORIENTED_EDGE ( 'NONE', *, *, #42529, .F. ) ;
#51860=DIRECTION ( 'NONE',  ( 0.000000000000000000, 0.000000000000000000, 1.000000000000000000 ) ) ;
#52023=ORIENTED_EDGE ( 'NONE', *, *, #102359, .T. ) ;
#52043=ORIENTED_EDGE ( 'NONE', *, *, #83840, .T. ) ;
#52209=EDGE_CURVE ( 'NONE', #188443, #27470, #164734, .T. ) ;
#52275=ORIENTED_EDGE ( 'NONE', *, *, #143324, .F. ) ;
#52321=PRODUCT_DEFINITION ( 'UNKNOWN', '', #134078, #159563 ) ;
#52434=DIRECTION ( 'NONE',  ( -0.1178549842436478201, -0.9930308165857339997, 7.149051953565419487E-31 ) ) ;
#52445=EDGE_CURVE ( 'NONE', #101229, #92045, #62760, .T. ) ;
#52474=CARTESIAN_POINT ( 'NONE',  ( -26.55135571139931727, -29.92032432623640048, -6.154557619715507855 ) ) ;
#52497=DIRECTION ( 'NONE',  ( 0.000000000000000000, 0.000000000000000000, -1.000000000000000000 ) ) ;
#52560=EDGE_CURVE ( 'NONE', #192038, #65708, #4730, .T. ) ;
#52952=ORIENTED_EDGE ( 'NONE', *, *, #87523, .T. ) ;
#53169=EDGE_CURVE ( 'NONE', #159210, #127511, #130599, .T. ) ;
#53174=ADVANCED_FACE ( 'NONE', ( #120204 ), #107014, .T. ) ;
#53186=CARTESIAN_POINT ( 'NONE',  ( -0.3431728551240714742, -71.74905178543389184, -4.999999999999999112 ) ) ;
#53220=( GEOMETRIC_REPRESENTATION_CONTEXT ( 3 ) GLOBAL_UNCERTAINTY_ASSIGNED_CONTEXT ( ( #82277 ) ) GLOBAL_UNIT_ASSIGNED_CONTEXT ( ( #175872, #80855, #4010 ) ) REPRESENTATION_CONTEXT ( 'NONE', 'WORKASPACE' ) );
#53370=LINE ( 'NONE', #115048, #163532 ) ;
#53542=DIRECTION ( 'NONE',  ( -0.000000000000000000, -0.000000000000000000, -1.000000000000000000 ) ) ;
#53570=CIRCLE ( 'NONE', #47239, 1.000000000000000888 ) ;
#53977=AXIS2_PLACEMENT_3D ( 'NONE', #108639, #94456, #124807 ) ;
#54205=ORIENTED_EDGE ( 'NONE', *, *, #166153, .F. ) ;
#54229=CARTESIAN_POINT ( 'NONE',  ( -12.49999999999997691, -89.99999999999997158, 0.000000000000000000 ) ) ;
#54327=EDGE_CURVE ( 'NONE', #40834, #41630, #121085, .T. ) ;
#54470=VERTEX_POINT ( 'NONE', #67118 ) ;
#54551=CARTESIAN_POINT ( 'NONE',  ( -4.911121358187451425E-30, -78.67194367458512261, -13.00000000000000000 ) ) ;
#54614=DIRECTION ( 'NONE',  ( 0.000000000000000000, 0.000000000000000000, -1.000000000000000000 ) ) ;
#54657=DIRECTION ( 'NONE',  ( -1.000000000000000000, 0.000000000000000000, 0.000000000000000000 ) ) ;
#54784=AXIS2_PLACEMENT_3D ( 'NONE', #132148, #92596, #181659 ) ;
#54861=DIRECTION ( 'NONE',  ( -1.000000000000000000, 0.000000000000000000, 0.000000000000000000 ) ) ;
#54912=ORIENTED_EDGE ( 'NONE', *, *, #59429, .T. ) ;
#55170=ADVANCED_FACE ( 'NONE', ( #197466 ), #198450, .F. ) ;
#55264=DIRECTION ( 'NONE',  ( 1.000000000000000000, -2.686023446673766396E-15, 0.000000000000000000 ) ) ;
#55311=ADVANCED_FACE ( 'NONE', ( #14416 ), #168100, .T. ) ;
#55464=ADVANCED_FACE ( 'NONE', ( #121589 ), #11284, .T. ) ;
#55659=CARTESIAN_POINT ( 'NONE',  ( -69.65682714487590488, -71.74905178543390605, 8.936314941956774358E-29 ) ) ;
#55959=CARTESIAN_POINT ( 'NONE',  ( -17.33350041961992360, -36.05029215572399437, -9.440814067905872520 ) ) ;
#56107=CARTESIAN_POINT ( 'NONE',  ( 5.000000000000000888, -140.0000000000000000, -12.99999999999999645 ) ) ;
#56154=AXIS2_PLACEMENT_3D ( 'NONE', #176069, #175062, #4197 ) ;
#56212=CIRCLE ( 'NONE', #117546, 216.0437394197456342 ) ;
#56235=CIRCLE ( 'NONE', #169228, 69.99999999999998579 ) ;
#56279=ORIENTED_EDGE ( 'NONE', *, *, #118198, .F. ) ;
#56334=ORIENTED_EDGE ( 'NONE', *, *, #95040, .F. ) ;
#56430=CARTESIAN_POINT ( 'NONE',  ( 69.65682714487590488, -71.74905178543389184, -13.00000000000000000 ) ) ;
#56448=ORIENTED_EDGE ( 'NONE', *, *, #40967, .T. ) ;
#56634=AXIS2_PLACEMENT_3D ( 'NONE', #129071, #146245, #39085 ) ;
#56988=CARTESIAN_POINT ( 'NONE',  ( 2.973862142520690366, -93.04182470242774627, -13.00000000000000000 ) ) ;
#57070=CIRCLE ( 'NONE', #195929, 2.649999999999999911 ) ;
#57076=CARTESIAN_POINT ( 'NONE',  ( -2.649999999999999911, -165.0000000000000000, -15.00000000000000000 ) ) ;
#57099=CARTESIAN_POINT ( 'NONE',  ( -11.30153831258470731, -188.0000000000000000, -15.00000000000000000 ) ) ;
#57122=CARTESIAN_POINT ( 'NONE',  ( 11.23596569267287038, -38.39307213609681213, -14.62819055234737320 ) ) ;
#57173=EDGE_CURVE ( 'NONE', #40598, #132987, #40292, .T. ) ;
#57594=EDGE_CURVE ( 'NONE', #169095, #15380, #185608, .T. ) ;
#57604=CARTESIAN_POINT ( 'NONE',  ( -27.86473085795038429, -131.0000000000000000, -13.99999999999999822 ) ) ;
#57612=AXIS2_PLACEMENT_3D ( 'NONE', #5235, #6237, #170648 ) ;
#57827=ORIENTED_EDGE ( 'NONE', *, *, #52445, .T. ) ;
#57917=ORIENTED_EDGE ( 'NONE', *, *, #44596, .T. ) ;
#57973=VERTEX_POINT ( 'NONE', #54229 ) ;
#58020=AXIS2_PLACEMENT_3D ( 'NONE', #154566, #94881, #187911 ) ;
#58029=ORIENTED_EDGE ( 'NONE', *, *, #47812, .T. ) ;
#58065=EDGE_CURVE ( 'NONE', #149173, #139926, #159900, .T. ) ;
#58351=AXIS2_PLACEMENT_3D ( 'NONE', #193468, #149956, #119624 ) ;
#58428=FACE_BOUND ( 'NONE', #8317, .T. ) ;
#59042=SURFACE_STYLE_USAGE ( .BOTH. , #62006 ) ;
#59409=FACE_BOUND ( 'NONE', #161919, .T. ) ;
#59417=VERTEX_POINT ( 'NONE', #56988 ) ;
#59429=EDGE_CURVE ( 'NONE', #54470, #118125, #117655, .T. ) ;
#59459=CIRCLE ( 'NONE', #56154, 10.00000000000000178 ) ;
#59498=ORIENTED_EDGE ( 'NONE', *, *, #8310, .T. ) ;
#59702=ORIENTED_EDGE ( 'NONE', *, *, #166248, .T. ) ;
#59719=AXIS2_PLACEMENT_3D ( 'NONE', #22381, #188252, #84031 ) ;
#59840=AXIS2_PLACEMENT_3D ( 'NONE', #23213, #190067, #65712 ) ;
#59958=EDGE_CURVE ( 'NONE', #43824, #40357, #115065, .T. ) ;
#60108=ORIENTED_EDGE ( 'NONE', *, *, #52560, .T. ) ;
#60138=ORIENTED_EDGE ( 'NONE', *, *, #124070, .F. ) ;
#60158=DIRECTION ( 'NONE',  ( 0.000000000000000000, 0.000000000000000000, -1.000000000000000000 ) ) ;
#60209=VERTEX_POINT ( 'NONE', #123595 ) ;
#60398=CARTESIAN_POINT ( 'NONE',  ( 9.352457526187951330E-15, -64.84118668444963873, -15.00000000000000000 ) ) ;
#60441=DIRECTION ( 'NONE',  ( 0.000000000000000000, 0.000000000000000000, 1.000000000000000000 ) ) ;
#60587=AXIS2_PLACEMENT_3D ( 'NONE', #165193, #88328, #150019 ) ;
#60618=AXIS2_PLACEMENT_3D ( 'NONE', #106066, #15059, #166772 ) ;
#60720=CARTESIAN_POINT ( 'NONE',  ( 5.000000000000000888, -130.0000000000000000, -13.99999999999999822 ) ) ;
#60740=LINE ( 'NONE', #166957, #199177 ) ;
#60759=AXIS2_PLACEMENT_3D ( 'NONE', #111368, #33538, #83012 ) ;
#60782=EDGE_CURVE ( 'NONE', #66675, #151273, #57070, .T. ) ;
#60938=DIRECTION ( 'NONE',  ( -1.000000000000000000, 0.000000000000000000, 0.000000000000000000 ) ) ;
#60997=APPLICATION_CONTEXT ( 'automotive_design' ) ;
#61133=AXIS2_PLACEMENT_3D ( 'NONE', #104325, #118510, #167981 ) ;
#61143=DIRECTION ( 'NONE',  ( -1.000000000000000000, 0.000000000000000000, 0.000000000000000000 ) ) ;
#61448=ADVANCED_FACE ( 'NONE', ( #3248 ), #145743, .F. ) ;
#61449=DIRECTION ( 'NONE',  ( -0.1178549842436472511, 0.9930308165857339997, -0.000000000000000000 ) ) ;
#61895=DIRECTION ( 'NONE',  ( 0.000000000000000000, 0.000000000000000000, -1.000000000000000000 ) ) ;
#61936=CARTESIAN_POINT ( 'NONE',  ( -2.973862142520652174, -93.04182470242764680, -4.999999999999999112 ) ) ;
#62006=SURFACE_SIDE_STYLE ('',( #164259 ) ) ;
#62026=DIRECTION ( 'NONE',  ( -0.000000000000000000, -0.000000000000000000, 1.000000000000000000 ) ) ;
#62256=CIRCLE ( 'NONE', #10632, 8.000000000000000000 ) ;
#62452=PLANE ( 'NONE',  #89925 ) ;
#62612=EDGE_CURVE ( 'NONE', #118125, #8593, #5354, .T. ) ;
#62760=CIRCLE ( 'NONE', #1425, 61.99999999999998579 ) ;
#62761=DIRECTION ( 'NONE',  ( -0.3041824702427698979, 0.9526137857479317628, 7.149051953565419487E-31 ) ) ;
#62894=DIRECTION ( 'NONE',  ( 5.392603844284257652E-33, -1.000000000000000000, 0.000000000000000000 ) ) ;
#62915=LINE ( 'NONE', #49746, #139856 ) ;
#63253=LINE ( 'NONE', #124933, #140791 ) ;
#63303=CIRCLE ( 'NONE', #176320, 10.00000000000000000 ) ;
#63484=CARTESIAN_POINT ( 'NONE',  ( -4.429638872090642462E-30, -165.0000000000000000, -13.00000000000000000 ) ) ;
#63491=ADVANCED_FACE ( 'NONE', ( #134357 ), #164690, .T. ) ;
#63554=CARTESIAN_POINT ( 'NONE',  ( 17.34328899321214124, -36.04909658921342697, -9.447446616692788623 ) ) ;
#63651=EDGE_CURVE ( 'NONE', #174040, #151167, #144348, .T. ) ;
#64134=EDGE_CURVE ( 'NONE', #133361, #12036, #187578, .T. ) ;
#64290=VERTEX_POINT ( 'NONE', #171397 ) ;
#64453=DIRECTION ( 'NONE',  ( -1.000000000000000000, 4.336808689942018352E-17, 0.000000000000000000 ) ) ;
#64493=AXIS2_PLACEMENT_3D ( 'NONE', #127492, #16357, #143654 ) ;
#64671=CARTESIAN_POINT ( 'NONE',  ( -14.65771419798590181, -37.23161142520606148, -13.64780077568128291 ) ) ;
#64859=DIRECTION ( 'NONE',  ( -4.336808689942018352E-17, 1.000000000000000000, 0.000000000000000000 ) ) ;
#64962=EDGE_CURVE ( 'NONE', #193517, #38038, #21682, .T. ) ;
#65094=EDGE_CURVE ( 'NONE', #12036, #149173, #34859, .T. ) ;
#65286=CARTESIAN_POINT ( 'NONE',  ( 20.76454096204583166, -34.24119976882402483, -10.56784353604181881 ) ) ;
#65353=FACE_OUTER_BOUND ( 'NONE', #149535, .T. ) ;
#65384=CARTESIAN_POINT ( 'NONE',  ( 11.30153831258471797, -180.0000000000000000, -4.999999999999999112 ) ) ;
#65677=DIRECTION ( 'NONE',  ( 0.9930308165857338887, 0.1178549842436482642, 0.000000000000000000 ) ) ;
#65678=DIRECTION ( 'NONE',  ( 0.000000000000000000, 0.000000000000000000, -1.000000000000000000 ) ) ;
#65708=VERTEX_POINT ( 'NONE', #158710 ) ;
#65712=DIRECTION ( 'NONE',  ( -1.000000000000000000, 0.000000000000000000, -5.421010862427521184E-16 ) ) ;
#65754=EDGE_CURVE ( 'NONE', #40357, #98984, #11911, .T. ) ;
#65762=FACE_OUTER_BOUND ( 'NONE', #87029, .T. ) ;
#65939=AXIS2_PLACEMENT_3D ( 'NONE', #94030, #155710, #17206 ) ;
#66136=AXIS2_PLACEMENT_3D ( 'NONE', #96297, #16501, #81120 ) ;
#66381=DIRECTION ( 'NONE',  ( -0.9930308165857338887, 0.1178549842436489581, 0.000000000000000000 ) ) ;
#66675=VERTEX_POINT ( 'NONE', #164722 ) ;
#66685=SHAPE_REPRESENTATION_RELATIONSHIP ( 'NONE' , 'NONE' ,  #85690, #189513 ) ;
#66709=EDGE_CURVE ( 'NONE', #155176, #57973, #121697, .T. ) ;
#66836=ORIENTED_EDGE ( 'NONE', *, *, #132163, .F. ) ;
#66850=VECTOR ( 'NONE', #35850, 1000.000000000000000 ) ;
#66959=DIRECTION ( 'NONE',  ( -1.000000000000000000, 5.392603844284257652E-33, 0.000000000000000000 ) ) ;
#67029=CYLINDRICAL_SURFACE ( 'NONE', #153598, 61.99999999999998579 ) ;
#67118=CARTESIAN_POINT ( 'NONE',  ( -19.97888994334923751, -34.65319547504295628, -4.999999999999999112 ) ) ;
#67143=CARTESIAN_POINT ( 'NONE',  ( 21.23184647844211881, -181.1785498424364675, -15.00000000000000000 ) ) ;
#67249=CIRCLE ( 'NONE', #167451, 61.99999999999998579 ) ;
#67375=ORIENTED_EDGE ( 'NONE', *, *, #166248, .F. ) ;
#67389=CARTESIAN_POINT ( 'NONE',  ( -5.000000000000000888, -130.0000000000000000, -13.99999999999999822 ) ) ;
#67615=CARTESIAN_POINT ( 'NONE',  ( 19.24578484527059175, -180.9428398739492820, -4.999999999999999112 ) ) ;
#67643=CARTESIAN_POINT ( 'NONE',  ( -15.58352941493655131, -36.85276851793626207, -13.27801782995927660 ) ) ;
#67681=SURFACE_STYLE_FILL_AREA ( #160692 ) ;
#67705=DIRECTION ( 'NONE',  ( -1.000000000000000000, 0.000000000000000000, 0.000000000000000000 ) ) ;
#67764=CARTESIAN_POINT ( 'NONE',  ( 193.3062444957835453, -155.7167183371837496, -4.999999999999999112 ) ) ;
#67851=CARTESIAN_POINT ( 'NONE',  ( 5.000000000000000888, -129.0000000000000000, -13.99999999999999822 ) ) ;
#67962=B_SPLINE_CURVE_WITH_KNOTS ( 'NONE', 3,
 ( #49138, #157307, #113764, #36931, #98593, #126945, #80449, #142122, #160287, #3607, #65286, #111792, #173480, #34953, #158294, #19783, #73296, #9619, #57122, #25798, #87444, #162283 ),
 .UNSPECIFIED., .F., .F.,
 ( 4, 2, 2, 2, 2, 2, 2, 2, 2, 2, 4 ),
 ( -3.098386792753634396E-05, 0.0007621651712067583836, 0.001555314210341053084, 0.003141612288609643786, 0.006314208445146832563, 0.01265940075822121792, 0.01583199691475840887, 0.01900459307129559808, 0.02059089114956419789, 0.02217718922783280117, 0.02534978538437000078 ),
 .UNSPECIFIED. ) ;
#67991=CIRCLE ( 'NONE', #164886, 206.0437394197456911 ) ;
#68108=CARTESIAN_POINT ( 'NONE',  ( -12.49999999999997691, -89.99999999999997158, -4.999999999999999112 ) ) ;
#68422=CYLINDRICAL_SURFACE ( 'NONE', #83405, 10.00000000000000178 ) ;
#68610=EDGE_CURVE ( 'NONE', #150223, #30088, #92827, .T. ) ;
#68639=CARTESIAN_POINT ( 'NONE',  ( -27.04846034099724505, -29.46915111869712334, -5.722710424963890929 ) ) ;
#68649=CARTESIAN_POINT ( 'NONE',  ( 2.995967610389833449E-15, -78.64189009824762877, -14.99999966871768642 ) ) ;
#68684=ORIENTED_EDGE ( 'NONE', *, *, #43478, .F. ) ;
#68699=CARTESIAN_POINT ( 'NONE',  ( -12.73749492396214578, -155.7167183371837496, -15.00000000000000000 ) ) ;
#68925=ORIENTED_EDGE ( 'NONE', *, *, #132407, .T. ) ;
#68983=EDGE_CURVE ( 'NONE', #149173, #122541, #104927, .T. ) ;
#69040=CIRCLE ( 'NONE', #114198, 2.649999999999999911 ) ;
#69242=DIRECTION ( 'NONE',  ( -1.000000000000000000, 0.000000000000000000, 0.000000000000000000 ) ) ;
#69262=EDGE_LOOP ( 'NONE', ( #14670, #27198, #71458 ) ) ;
#69472=EDGE_CURVE ( 'NONE', #161389, #94667, #34219, .T. ) ;
#69568=EDGE_CURVE ( 'NONE', #27470, #116009, #192870, .T. ) ;
#69843=ORIENTED_EDGE ( 'NONE', *, *, #107568, .T. ) ;
#69890=CIRCLE ( 'NONE', #182914, 8.000000000000000000 ) ;
#69993=ORIENTED_EDGE ( 'NONE', *, *, #52209, .F. ) ;
#70139=ORIENTED_EDGE ( 'NONE', *, *, #68610, .F. ) ;
#70507=VERTEX_POINT ( 'NONE', #78189 ) ;
#70632=EDGE_CURVE ( 'NONE', #159210, #150536, #196229, .T. ) ;
#70667=FACE_OUTER_BOUND ( 'NONE', #176575, .T. ) ;
#70675=ORIENTED_EDGE ( 'NONE', *, *, #65094, .T. ) ;
#70680=DIRECTION ( 'NONE',  ( -1.000000000000000000, 0.000000000000000000, 0.000000000000000000 ) ) ;
#70723=DIRECTION ( 'NONE',  ( 0.000000000000000000, 0.000000000000000000, 1.000000000000000000 ) ) ;
#70811=CARTESIAN_POINT ( 'NONE',  ( -7.652493125987827050, -39.26116846142902261, -15.00000000000000000 ) ) ;
#71026=DIRECTION ( 'NONE',  ( -1.000000000000000000, -4.336808689942018352E-17, 3.574525976782710181E-31 ) ) ;
#71161=EDGE_CURVE ( 'NONE', #33072, #97924, #44359, .T. ) ;
#71458=ORIENTED_EDGE ( 'NONE', *, *, #88386, .F. ) ;
#71687=EDGE_LOOP ( 'NONE', ( #161897, #10237, #194813, #98215 ) ) ;
#71707=CARTESIAN_POINT ( 'NONE',  ( 5.000000000000001776, -120.0000000000000142, -15.00000000000000000 ) ) ;
#71876=DIRECTION ( 'NONE',  ( 0.000000000000000000, 0.000000000000000000, 1.000000000000000000 ) ) ;
#71984=ORIENTED_EDGE ( 'NONE', *, *, #69472, .T. ) ;
#71985=CARTESIAN_POINT ( 'NONE',  ( 19.24578484527059175, -180.9428398739492820, -1.787262988391354872E-28 ) ) ;
#72162=EDGE_LOOP ( 'NONE', ( #132311, #82652, #43273, #183903 ) ) ;
#72556=EDGE_CURVE ( 'NONE', #27838, #59417, #151032, .T. ) ;
#72669=DIRECTION ( 'NONE',  ( -0.000000000000000000, -0.000000000000000000, 1.000000000000000000 ) ) ;
#72682=DIRECTION ( 'NONE',  ( 1.000000000000000000, 0.000000000000000000, 0.000000000000000000 ) ) ;
#72778=LINE ( 'NONE', #57604, #80916 ) ;
#72809=AXIS2_PLACEMENT_3D ( 'NONE', #164101, #167081, #150925 ) ;
#73148=CARTESIAN_POINT ( 'NONE',  ( -19.97888994334928014, -34.65319547504296338, -5.175670227483850638 ) ) ;
#73296=CARTESIAN_POINT ( 'NONE',  ( 12.73189700295822213, -37.92323000020837753, -14.26360274717254129 ) ) ;
#73522=ORIENTED_EDGE ( 'NONE', *, *, #157036, .T. ) ;
#73639=CYLINDRICAL_SURFACE ( 'NONE', #144978, 8.000000000000000000 ) ;
#73681=EDGE_CURVE ( 'NONE', #99125, #49756, #199432, .T. ) ;
#73738=ORIENTED_EDGE ( 'NONE', *, *, #139548, .T. ) ;
#73781=AXIS2_PLACEMENT_3D ( 'NONE', #110945, #64453, #129083 ) ;
#73972=DIRECTION ( 'NONE',  ( 1.000000000000000000, -4.336808689942018352E-17, 0.000000000000000000 ) ) ;
#74080=ORIENTED_EDGE ( 'NONE', *, *, #182203, .F. ) ;
#74166=VERTEX_POINT ( 'NONE', #48735 ) ;
#74305=CIRCLE ( 'NONE', #45274, 8.000000000000000000 ) ;
#74322=ORIENTED_EDGE ( 'NONE', *, *, #93154, .F. ) ;
#74330=CIRCLE ( 'NONE', #77479, 69.99999999999997158 ) ;
#74509=PLANE ( 'NONE',  #127534 ) ;
#74605=ORIENTED_EDGE ( 'NONE', *, *, #38962, .T. ) ;
#74607=ORIENTED_EDGE ( 'NONE', *, *, #142789, .F. ) ;
#74851=EDGE_CURVE ( 'NONE', #169095, #22637, #40543, .T. ) ;
#74935=CARTESIAN_POINT ( 'NONE',  ( -193.3062444957834884, -155.7167183371838064, -15.00000000000000000 ) ) ;
#75145=EDGE_LOOP ( 'NONE', ( #181565, #105697, #36494 ) ) ;
#75423=FACE_OUTER_BOUND ( 'NONE', #142552, .T. ) ;
#75643=DIRECTION ( 'NONE',  ( 4.336808689942018352E-17, -1.000000000000000000, 0.000000000000000000 ) ) ;
#75655=AXIS2_PLACEMENT_3D ( 'NONE', #189718, #177550, #39019 ) ;
#75703=CIRCLE ( 'NONE', #46706, 206.0437394197456342 ) ;
#75726=CARTESIAN_POINT ( 'NONE',  ( -5.000000000000000888, -129.0000000000000000, -13.99999999999999822 ) ) ;
#75787=CYLINDRICAL_SURFACE ( 'NONE', #167704, 8.000000000000000000 ) ;
#75803=ORIENTED_EDGE ( 'NONE', *, *, #83344, .F. ) ;
#76196=LINE ( 'NONE', #153035, #170967 ) ;
#76282=DIRECTION ( 'NONE',  ( 0.000000000000000000, 0.000000000000000000, 1.000000000000000000 ) ) ;
#76488=VECTOR ( 'NONE', #198276, 1000.000000000000000 ) ;
#76671=VECTOR ( 'NONE', #147449, 1000.000000000000000 ) ;
#76723=CARTESIAN_POINT ( 'NONE',  ( 19.60416288135285967, -34.86663519103794329, -6.666020143318704072 ) ) ;
#76887=DIRECTION ( 'NONE',  ( 0.000000000000000000, -1.000000000000000000, 0.000000000000000000 ) ) ;
#76922=FACE_OUTER_BOUND ( 'NONE', #13996, .T. ) ;
#77336=ORIENTED_EDGE ( 'NONE', *, *, #97058, .F. ) ;
#77384=DIRECTION ( 'NONE',  ( -1.000000000000000000, 5.392603844284257652E-33, 0.000000000000000000 ) ) ;
#77444=VECTOR ( 'NONE', #51200, 1000.000000000000000 ) ;
#77479=AXIS2_PLACEMENT_3D ( 'NONE', #131326, #143489, #193014 ) ;
#77649=ORIENTED_EDGE ( 'NONE', *, *, #48243, .F. ) ;
#77720=CARTESIAN_POINT ( 'NONE',  ( 17.83380816373549038, -35.80792897213662940, -9.022620566401460707 ) ) ;
#77828=EDGE_CURVE ( 'NONE', #59417, #165210, #199477, .T. ) ;
#77881=ORIENTED_EDGE ( 'NONE', *, *, #22446, .T. ) ;
#77925=DIRECTION ( 'NONE',  ( -0.9526137857479314297, -0.3041824702427711746, 0.000000000000000000 ) ) ;
#78080=LINE ( 'NONE', #126572, #1017 ) ;
#78109=ORIENTED_EDGE ( 'NONE', *, *, #77828, .T. ) ;
#78189=CARTESIAN_POINT ( 'NONE',  ( -19.24578484527059175, -180.9428398739491684, 1.787262988391354872E-28 ) ) ;
#78348=ORIENTED_EDGE ( 'NONE', *, *, #73681, .T. ) ;
#78587=EDGE_CURVE ( 'NONE', #142920, #164159, #141253, .T. ) ;
#78615=DIRECTION ( 'NONE',  ( -5.392603844284257652E-33, -1.000000000000000000, -0.000000000000000000 ) ) ;
#78771=CARTESIAN_POINT ( 'NONE',  ( -11.30153831258470731, -188.0000000000000000, 0.000000000000000000 ) ) ;
#78840=ORIENTED_EDGE ( 'NONE', *, *, #5261, .F. ) ;
#78859=DIRECTION ( 'NONE',  ( -1.000000000000000000, 5.392603844284257652E-33, -0.000000000000000000 ) ) ;
#78941=CARTESIAN_POINT ( 'NONE',  ( -19.99999999999998224, -180.0000000000000000, -4.999999999999999112 ) ) ;
#79002=CARTESIAN_POINT ( 'NONE',  ( 2.285367203649815956E-16, -78.65850330665435308, -13.00000000000000000 ) ) ;
#79148=EDGE_CURVE ( 'NONE', #184761, #137566, #2600, .T. ) ;
#79163=CIRCLE ( 'NONE', #172718, 10.00000000000000355 ) ;
#79169=DIRECTION ( 'NONE',  ( 0.000000000000000000, 0.000000000000000000, 1.000000000000000000 ) ) ;
#79382=ORIENTED_EDGE ( 'NONE', *, *, #103239, .T. ) ;
#79551=CARTESIAN_POINT ( 'NONE',  ( 11.30153831258470731, -180.0000000000000000, 0.000000000000000000 ) ) ;
#79554=AXIS2_PLACEMENT_3D ( 'NONE', #50279, #157452, #140278 ) ;
#79600=DIRECTION ( 'NONE',  ( -1.000000000000000000, 0.000000000000000000, 0.000000000000000000 ) ) ;
#79645=EDGE_LOOP ( 'NONE', ( #14379, #119836, #126598, #131941, #24352, #87609, #56334, #26924 ) ) ;
#79930=DIRECTION ( 'NONE',  ( 0.9526137857479317628, 0.3041824702427701199, 0.000000000000000000 ) ) ;
#79976=CARTESIAN_POINT ( 'NONE',  ( 22.73749492396215288, -155.7167183371838064, 0.000000000000000000 ) ) ;
#80056=CARTESIAN_POINT ( 'NONE',  ( -9.656827144875922642, -71.74905178543390605, -4.999999999999999112 ) ) ;
#80374=FACE_OUTER_BOUND ( 'NONE', #192669, .T. ) ;
#80409=CARTESIAN_POINT ( 'NONE',  ( -7.652493125962417153, -39.26116846143397510, -13.00000000000000000 ) ) ;
#80449=CARTESIAN_POINT ( 'NONE',  ( 26.21537839388344793, -30.21513421080428685, -6.441064297728048338 ) ) ;
#80619=SHAPE_DEFINITION_REPRESENTATION ( #156746, #85690 ) ;
#80818=CARTESIAN_POINT ( 'NONE',  ( -11.23589665953924666, -38.39309219976287579, -14.62820445599025199 ) ) ;
#80845=ORIENTED_EDGE ( 'NONE', *, *, #179869, .T. ) ;
#80850=DIRECTION ( 'NONE',  ( 0.000000000000000000, 0.000000000000000000, -1.000000000000000000 ) ) ;
#80855=( NAMED_UNIT ( * ) PLANE_ANGLE_UNIT ( ) SI_UNIT ( $, .RADIAN. ) );
#80866=CARTESIAN_POINT ( 'NONE',  ( 2.649999999999999911, -105.0000000000000000, -15.00000000000000000 ) ) ;
#80916=VECTOR ( 'NONE', #181939, 1000.000000000000000 ) ;
#81120=DIRECTION ( 'NONE',  ( 6.938893903907222461E-16, -1.000000000000000000, 0.000000000000000000 ) ) ;
#81293=DIRECTION ( 'NONE',  ( 0.000000000000000000, 0.000000000000000000, -1.000000000000000000 ) ) ;
#81311=ADVANCED_FACE ( 'NONE', ( #83076 ), #117425, .F. ) ;
#81317=ORIENTED_EDGE ( 'NONE', *, *, #21840, .F. ) ;
#81451=ADVANCED_FACE ( 'NONE', ( #163950 ), #143754, .F. ) ;
#81671=CARTESIAN_POINT ( 'NONE',  ( 13.16545937439093272, -37.77263716084178213, -11.88623523016686967 ) ) ;
#81729=CARTESIAN_POINT ( 'NONE',  ( 10.59477242850415024, -90.60836494048558620, 0.000000000000000000 ) ) ;
#81856=AXIS2_PLACEMENT_3D ( 'NONE', #9000, #118171, #179862 ) ;
#81939=ADVANCED_FACE ( 'NONE', ( #10262 ), #62452, .F. ) ;
#82054=AXIS2_PLACEMENT_3D ( 'NONE', #82060, #99242, #83075 ) ;
#82060=CARTESIAN_POINT ( 'NONE',  ( 0.000000000000000000, 0.000000000000000000, 0.000000000000000000 ) ) ;
#82197=MECHANICAL_DESIGN_GEOMETRIC_PRESENTATION_REPRESENTATION('',(#179109),#33882);
#82248=ORIENTED_EDGE ( 'NONE', *, *, #50678, .F. ) ;
#82277=UNCERTAINTY_MEASURE_WITH_UNIT (LENGTH_MEASURE( 1.000000000000000082E-05 ), #175872, 'distance_accuracy_value', 'NONE');
#82280=AXIS2_PLACEMENT_3D ( 'NONE', #164983, #26478, #197311 ) ;
#82288=EDGE_CURVE ( 'NONE', #6627, #145279, #115764, .T. ) ;
#82498=AXIS2_PLACEMENT_3D ( 'NONE', #82529, #144211, #8454 ) ;
#82511=DIRECTION ( 'NONE',  ( 1.000000000000000000, -4.336808689942018352E-17, 0.000000000000000000 ) ) ;
#82529=CARTESIAN_POINT ( 'NONE',  ( 7.992609269207028790E-30, -165.0000000000000000, -15.00000000000000000 ) ) ;
#82652=ORIENTED_EDGE ( 'NONE', *, *, #38347, .T. ) ;
#82837=( LENGTH_UNIT ( ) NAMED_UNIT ( * ) SI_UNIT ( .MILLI., .METRE. ) );
#82917=EDGE_CURVE ( 'NONE', #54470, #169095, #67249, .T. ) ;
#83012=DIRECTION ( 'NONE',  ( 0.000000000000000000, -1.000000000000000000, 0.000000000000000000 ) ) ;
#83028=FACE_OUTER_BOUND ( 'NONE', #114384, .T. ) ;
#83033=CARTESIAN_POINT ( 'NONE',  ( 193.3062444957835453, -155.7167183371837496, -15.00000000000000000 ) ) ;
#83075=DIRECTION ( 'NONE',  ( 1.000000000000000000, 0.000000000000000000, 0.000000000000000000 ) ) ;
#83076=FACE_OUTER_BOUND ( 'NONE', #102499, .T. ) ;
#83082=ORIENTED_EDGE ( 'NONE', *, *, #65754, .F. ) ;
#83140=AXIS2_PLACEMENT_3D ( 'NONE', #125701, #140861, #29727 ) ;
#83344=EDGE_CURVE ( 'NONE', #38038, #149173, #189948, .T. ) ;
#83386=DIRECTION ( 'NONE',  ( -1.000000000000000000, 0.000000000000000000, 0.000000000000000000 ) ) ;
#83405=AXIS2_PLACEMENT_3D ( 'NONE', #37089, #96755, #98748 ) ;
#83531=EDGE_LOOP ( 'NONE', ( #31652, #83082, #131510, #66836 ) ) ;
#83609=ORIENTED_EDGE ( 'NONE', *, *, #97135, .T. ) ;
#83641=AXIS2_PLACEMENT_3D ( 'NONE', #171074, #155897, #17395 ) ;
#83757=CARTESIAN_POINT ( 'NONE',  ( -2.973862142520662832, -93.04182470242767522, -15.00000000000000000 ) ) ;
#83840=EDGE_CURVE ( 'NONE', #98984, #132746, #118962, .T. ) ;
#83864=DIRECTION ( 'NONE',  ( 1.000000000000000000, 0.000000000000000000, 0.000000000000000000 ) ) ;
#84031=DIRECTION ( 'NONE',  ( 1.000000000000000000, 0.000000000000000000, 0.000000000000000000 ) ) ;
#84050=EDGE_CURVE ( 'NONE', #98984, #133568, #12455, .T. ) ;
#84136=ORIENTED_EDGE ( 'NONE', *, *, #113277, .T. ) ;
#84395=CARTESIAN_POINT ( 'NONE',  ( -4.429638872090642462E-30, -165.0000000000000000, -13.00000000000000000 ) ) ;
#84595=ADVANCED_FACE ( 'NONE', ( #191773 ), #68422, .T. ) ;
#84673=CARTESIAN_POINT ( 'NONE',  ( 15.76494486619527180, -36.76728419955058058, -10.58017208825962818 ) ) ;
#84711=EDGE_CURVE ( 'NONE', #167341, #99125, #28615, .T. ) ;
#84805=CARTESIAN_POINT ( 'NONE',  ( 2.995967610389833449E-15, -78.62686331009497565, -14.99999901254159873 ) ) ;
#85422=EDGE_LOOP ( 'NONE', ( #31538, #190304, #73522, #195984 ) ) ;
#85543=VECTOR ( 'NONE', #191850, 1000.000000000000000 ) ;
#85690=SHAPE_REPRESENTATION ( 'front house', ( #82054 ), #50057 ) ;
#85773=ORIENTED_EDGE ( 'NONE', *, *, #168827, .T. ) ;
#85865=DIRECTION ( 'NONE',  ( -0.000000000000000000, -0.000000000000000000, 1.000000000000000000 ) ) ;
#85907=CIRCLE ( 'NONE', #131222, 40.00000000000002132 ) ;
#85951=DIRECTION ( 'NONE',  ( -1.000000000000000000, 0.000000000000000000, 0.000000000000000000 ) ) ;
#85978=EDGE_CURVE ( 'NONE', #14496, #145279, #153236, .T. ) ;
#86029=ORIENTED_EDGE ( 'NONE', *, *, #175799, .F. ) ;
#86075=DIRECTION ( 'NONE',  ( 0.000000000000000000, 0.000000000000000000, 1.000000000000000000 ) ) ;
#86153=ORIENTED_EDGE ( 'NONE', *, *, #64134, .F. ) ;
#86185=FACE_OUTER_BOUND ( 'NONE', #113563, .T. ) ;
#86268=ORIENTED_EDGE ( 'NONE', *, *, #52445, .F. ) ;
#86325=ORIENTED_EDGE ( 'NONE', *, *, #103239, .F. ) ;
#86762=DIRECTION ( 'NONE',  ( 0.000000000000000000, 0.000000000000000000, 1.000000000000000000 ) ) ;
#86767=DIRECTION ( 'NONE',  ( 0.000000000000000000, 0.000000000000000000, -1.000000000000000000 ) ) ;
#86791=DIRECTION ( 'NONE',  ( 1.000000000000000000, -5.392603844284257652E-33, 0.000000000000000000 ) ) ;
#86823=LINE ( 'NONE', #180858, #184009 ) ;
#87029=EDGE_LOOP ( 'NONE', ( #20401, #28497, #155691, #197144 ) ) ;
#87089=ORIENTED_EDGE ( 'NONE', *, *, #152778, .T. ) ;
#87155=AXIS2_PLACEMENT_3D ( 'NONE', #197996, #72669, #178854 ) ;
#87247=ORIENTED_EDGE ( 'NONE', *, *, #189313, .F. ) ;
#87296=CARTESIAN_POINT ( 'NONE',  ( -14.06429661546934184, -37.45132032961591761, -11.50520302883531087 ) ) ;
#87315=DIRECTION ( 'NONE',  ( -0.000000000000000000, -0.000000000000000000, 1.000000000000000000 ) ) ;
#87444=CARTESIAN_POINT ( 'NONE',  ( 8.695259559498534685, -39.05792023227123622, -15.00000000000000178 ) ) ;
#87523=EDGE_CURVE ( 'NONE', #133568, #60209, #17726, .T. ) ;
#87609=ORIENTED_EDGE ( 'NONE', *, *, #189313, .T. ) ;
#87663=ORIENTED_EDGE ( 'NONE', *, *, #34170, .F. ) ;
#87760=DIRECTION ( 'NONE',  ( -1.000000000000000000, 5.392603844284257652E-33, 0.000000000000000000 ) ) ;
#87766=ORIENTED_EDGE ( 'NONE', *, *, #43996, .F. ) ;
#88003=SPHERICAL_SURFACE ( 'NONE', #44030, 8.000000000000000000 ) ;
#88328=DIRECTION ( 'NONE',  ( 0.000000000000000000, 0.000000000000000000, 1.000000000000000000 ) ) ;
#88386=EDGE_CURVE ( 'NONE', #164159, #133568, #135807, .T. ) ;
#88515=CARTESIAN_POINT ( 'NONE',  ( 193.3062444957835453, -155.7167183371837496, -4.999999999999999112 ) ) ;
#88604=DIRECTION ( 'NONE',  ( 1.000000000000000000, 0.000000000000000000, 0.000000000000000000 ) ) ;
#88982=DIRECTION ( 'NONE',  ( 1.000000000000000000, -5.392603844284257652E-33, 0.000000000000000000 ) ) ;
#89122=CARTESIAN_POINT ( 'NONE',  ( -27.86473085795038429, -130.0000000000000000, -13.99999999999999822 ) ) ;
#89281=CARTESIAN_POINT ( 'NONE',  ( -4.999999999999999112, -140.0000000000000000, -12.99999999999999645 ) ) ;
#89364=FACE_OUTER_BOUND ( 'NONE', #92070, .T. ) ;
#89567=EDGE_LOOP ( 'NONE', ( #4402, #31658, #116340, #51756 ) ) ;
#89760=DIRECTION ( 'NONE',  ( -1.000000000000000000, 0.000000000000000000, 0.000000000000000000 ) ) ;
#89789=DIRECTION ( 'NONE',  ( 0.000000000000000000, 0.000000000000000000, -1.000000000000000000 ) ) ;
#89802=DIRECTION ( 'NONE',  ( 1.000000000000000000, 0.000000000000000000, 0.000000000000000000 ) ) ;
#89815=DIRECTION ( 'NONE',  ( -1.000000000000000000, 0.000000000000000000, 0.000000000000000000 ) ) ;
#89925=AXIS2_PLACEMENT_3D ( 'NONE', #140294, #29170, #75643 ) ;
#90265=DIRECTION ( 'NONE',  ( 0.000000000000000000, 0.000000000000000000, -1.000000000000000000 ) ) ;
#90271=CARTESIAN_POINT ( 'NONE',  ( -19.78838472062539822, -34.76237422906578445, -6.192482694737989846 ) ) ;
#90345=CARTESIAN_POINT ( 'NONE',  ( 27.86273085795036408, -28.69962071417356242, -4.999999999999999112 ) ) ;
#90372=PRESENTATION_STYLE_ASSIGNMENT (( #59042 ) ) ;
#90464=CARTESIAN_POINT ( 'NONE',  ( -12.49999999999997691, -89.99999999999997158, -15.00000000000000000 ) ) ;
#90966=DIRECTION ( 'NONE',  ( 0.000000000000000000, 1.000000000000000000, 0.000000000000000000 ) ) ;
#91083=DIRECTION ( 'NONE',  ( 0.000000000000000000, 1.000000000000000000, 0.000000000000000000 ) ) ;
#91257=DIRECTION ( 'NONE',  ( 0.000000000000000000, 0.000000000000000000, -1.000000000000000000 ) ) ;
#91375=ORIENTED_EDGE ( 'NONE', *, *, #121465, .T. ) ;
#91731=DIRECTION ( 'NONE',  ( -1.000000000000000000, 0.000000000000000000, 0.000000000000000000 ) ) ;
#91768=AXIS2_PLACEMENT_3D ( 'NONE', #173884, #78859, #80850 ) ;
#91879=STYLED_ITEM ( 'NONE', ( #114169 ), #189513 ) ;
#91909=VECTOR ( 'NONE', #116219, 1000.000000000000000 ) ;
#91933=CARTESIAN_POINT ( 'NONE',  ( 11.30153831258470731, -190.0000000000000000, -4.999999999999999112 ) ) ;
#92002=CIRCLE ( 'NONE', #8023, 69.99999999999997158 ) ;
#92045=VERTEX_POINT ( 'NONE', #164782 ) ;
#92070=EDGE_LOOP ( 'NONE', ( #8438, #26124, #98109 ) ) ;
#92125=EDGE_CURVE ( 'NONE', #38038, #118785, #72778, .T. ) ;
#92237=DIRECTION ( 'NONE',  ( 0.000000000000000000, 0.000000000000000000, -1.000000000000000000 ) ) ;
#92353=CARTESIAN_POINT ( 'NONE',  ( -9.656827144875922642, -71.74905178543390605, -15.00000000000000000 ) ) ;
#92596=DIRECTION ( 'NONE',  ( 0.000000000000000000, 0.000000000000000000, -1.000000000000000000 ) ) ;
#92730=ADVANCED_FACE ( 'NONE', ( #127193, #17054, #126215, #32224 ), #125228, .T. ) ;
#92809=ORIENTED_EDGE ( 'NONE', *, *, #72556, .T. ) ;
#92827=CIRCLE ( 'NONE', #2326, 216.0437394197456342 ) ;
#92879=CARTESIAN_POINT ( 'NONE',  ( 19.11401883044621286, -35.13836984581306666, -7.540766371346785846 ) ) ;
#93154=EDGE_CURVE ( 'NONE', #92045, #159210, #163663, .T. ) ;
#93301=DIRECTION ( 'NONE',  ( 1.000000000000000000, 0.000000000000000000, 0.000000000000000000 ) ) ;
#93309=CIRCLE ( 'NONE', #83641, 206.0437394197456911 ) ;
#93340=CYLINDRICAL_SURFACE ( 'NONE', #114054, 214.0437394197456342 ) ;
#93430=ORIENTED_EDGE ( 'NONE', *, *, #102515, .T. ) ;
#93454=AXIS2_PLACEMENT_3D ( 'NONE', #107282, #180200, #119505 ) ;
#93839=CIRCLE ( 'NONE', #58351, 8.000000000000001776 ) ;
#94030=CARTESIAN_POINT ( 'NONE',  ( -11.30153831258471975, -180.0000000000000000, -4.999999999999999112 ) ) ;
#94170=CARTESIAN_POINT ( 'NONE',  ( 6.856101608890750167E-16, -78.63162257080495010, -12.99999901186700946 ) ) ;
#94248=TOROIDAL_SURFACE ( 'NONE', #149144, 69.99999999999998579, 10.00000000000000000 ) ;
#94456=DIRECTION ( 'NONE',  ( 0.000000000000000000, 0.000000000000000000, -1.000000000000000000 ) ) ;
#94534=CARTESIAN_POINT ( 'NONE',  ( 5.000000000000001776, -120.0000000000000142, -13.00000000000000000 ) ) ;
#94568=EDGE_CURVE ( 'NONE', #60209, #158522, #32170, .T. ) ;
#94667=VERTEX_POINT ( 'NONE', #170031 ) ;
#94873=AXIS2_PLACEMENT_3D ( 'NONE', #177588, #39055, #100713 ) ;
#94881=DIRECTION ( 'NONE',  ( 0.000000000000000000, 0.000000000000000000, -1.000000000000000000 ) ) ;
#94965=VECTOR ( 'NONE', #71876, 1000.000000000000000 ) ;
#95040=EDGE_CURVE ( 'NONE', #141411, #27838, #121047, .T. ) ;
#95065=DIRECTION ( 'NONE',  ( -1.000000000000000000, 0.000000000000000000, 0.000000000000000000 ) ) ;
#95210=AXIS2_PLACEMENT_3D ( 'NONE', #19537, #113517, #191369 ) ;
#95298=ORIENTED_EDGE ( 'NONE', *, *, #198923, .F. ) ;
#95324=AXIS2_PLACEMENT_3D ( 'NONE', #12933, #103939, #87760 ) ;
#95669=AXIS2_PLACEMENT_3D ( 'NONE', #144376, #190895, #114028 ) ;
#95742=DIRECTION ( 'NONE',  ( -1.000000000000000000, 5.392603844284257652E-33, -0.000000000000000000 ) ) ;
#95759=CARTESIAN_POINT ( 'NONE',  ( -19.97888994334924817, -34.65319547504297759, 0.000000000000000000 ) ) ;
#95794=ADVANCED_FACE ( 'NONE', ( #107115 ), #75787, .F. ) ;
#95856=ORIENTED_EDGE ( 'NONE', *, *, #170997, .F. ) ;
#95864=AXIS2_PLACEMENT_3D ( 'NONE', #9041, #85865, #8020 ) ;
#95927=CARTESIAN_POINT ( 'NONE',  ( 11.30153831258473573, -180.0000000000000284, -4.999999999999999112 ) ) ;
#96037=VERTEX_POINT ( 'NONE', #91933 ) ;
#96284=ORIENTED_EDGE ( 'NONE', *, *, #116598, .F. ) ;
#96287=ORIENTED_EDGE ( 'NONE', *, *, #167994, .T. ) ;
#96297=CARTESIAN_POINT ( 'NONE',  ( -11.30153831258471442, -180.0000000000000000, -4.999999999999999112 ) ) ;
#96410=DIRECTION ( 'NONE',  ( -1.000000000000000000, 5.392603844284257652E-33, 0.000000000000000000 ) ) ;
#96495=ORIENTED_EDGE ( 'NONE', *, *, #68610, .T. ) ;
#96625=CIRCLE ( 'NONE', #51327, 214.0437394197456342 ) ;
#96755=DIRECTION ( 'NONE',  ( 0.000000000000000000, 0.000000000000000000, 1.000000000000000000 ) ) ;
#96796=AXIS2_PLACEMENT_3D ( 'NONE', #25181, #135343, #120150 ) ;
#96981=CYLINDRICAL_SURFACE ( 'NONE', #102080, 8.000000000000000000 ) ;
#97058=EDGE_CURVE ( 'NONE', #137566, #41468, #180718, .T. ) ;
#97135=EDGE_CURVE ( 'NONE', #178033, #96037, #16009, .T. ) ;
#97541=CARTESIAN_POINT ( 'NONE',  ( -2.973862142520655727, -93.04182470242766101, -13.00000000000000000 ) ) ;
#97668=LINE ( 'NONE', #140215, #77444 ) ;
#97688=EDGE_LOOP ( 'NONE', ( #58029, #110895 ) ) ;
#97924=VERTEX_POINT ( 'NONE', #39241 ) ;
#97956=CARTESIAN_POINT ( 'NONE',  ( -17.38101740422981933, -36.03988305276040194, -12.45567487529643635 ) ) ;
#98109=ORIENTED_EDGE ( 'NONE', *, *, #132407, .F. ) ;
#98186=CIRCLE ( 'NONE', #59840, 8.000000000000001776 ) ;
#98215=ORIENTED_EDGE ( 'NONE', *, *, #52209, .T. ) ;
#98395=AXIS2_PLACEMENT_3D ( 'NONE', #123091, #126084, #110908 ) ;
#98428=CARTESIAN_POINT ( 'NONE',  ( -5.000000000000000000, -120.0000000000000142, -15.00000000000000000 ) ) ;
#98512=AXIS2_PLACEMENT_3D ( 'NONE', #39169, #100827, #99834 ) ;
#98593=CARTESIAN_POINT ( 'NONE',  ( 27.04875460227163586, -29.46888106016232811, -5.722453210188423789 ) ) ;
#98630=ORIENTED_EDGE ( 'NONE', *, *, #170373, .T. ) ;
#98748=DIRECTION ( 'NONE',  ( 1.000000000000000000, 0.000000000000000000, 0.000000000000000000 ) ) ;
#98842=CARTESIAN_POINT ( 'NONE',  ( 11.92298843706294420, -38.18315321023221287, -12.32826034376742363 ) ) ;
#98876=VECTOR ( 'NONE', #87315, 1000.000000000000000 ) ;
#98984=VERTEX_POINT ( 'NONE', #155790 ) ;
#99125=VERTEX_POINT ( 'NONE', #14299 ) ;
#99242=DIRECTION ( 'NONE',  ( 0.000000000000000000, 0.000000000000000000, 1.000000000000000000 ) ) ;
#99493=ORIENTED_EDGE ( 'NONE', *, *, #118963, .F. ) ;
#99672=CARTESIAN_POINT ( 'NONE',  ( 20.73749492396215288, -155.7167183371838064, 0.000000000000000000 ) ) ;
#99709=DIRECTION ( 'NONE',  ( 0.000000000000000000, 0.000000000000000000, -1.000000000000000000 ) ) ;
#99750=DIRECTION ( 'NONE',  ( -1.000000000000000000, 4.336808689942018352E-17, 0.000000000000000000 ) ) ;
#99773=PRODUCT_CONTEXT ( 'NONE', #110017, 'mechanical' ) ;
#99834=DIRECTION ( 'NONE',  ( -1.000000000000000000, 0.000000000000000000, 0.000000000000000000 ) ) ;
#99851=CARTESIAN_POINT ( 'NONE',  ( 7.652493125987820832, -39.26116846142902261, -13.00000000000000000 ) ) ;
#100031=ADVANCED_FACE ( 'NONE', ( #65762 ), #190116, .T. ) ;
#100435=FACE_OUTER_BOUND ( 'NONE', #34145, .T. ) ;
#100713=DIRECTION ( 'NONE',  ( -1.000000000000000000, 0.000000000000000000, 5.204170427930421283E-16 ) ) ;
#100827=DIRECTION ( 'NONE',  ( 0.000000000000000000, 0.000000000000000000, -1.000000000000000000 ) ) ;
#100961=EDGE_CURVE ( 'NONE', #165210, #23117, #32359, .T. ) ;
#101002=DIRECTION ( 'NONE',  ( 1.000000000000000000, -5.392603844284257652E-33, 0.000000000000000000 ) ) ;
#101008=DIRECTION ( 'NONE',  ( 0.000000000000000000, 1.000000000000000000, 0.000000000000000000 ) ) ;
#101123=DIRECTION ( 'NONE',  ( 0.000000000000000000, 0.000000000000000000, 1.000000000000000000 ) ) ;
#101161=ORIENTED_EDGE ( 'NONE', *, *, #130358, .T. ) ;
#101229=VERTEX_POINT ( 'NONE', #172863 ) ;
#101418=CLOSED_SHELL ( 'NONE', ( #130486, #394, #176759, #122577, #156437, #18328, #114410, #15156, #25330, #13706, #55464, #81939, #105243, #26668, #185767, #151408, #4808, #81311, #63491, #55311, #144876, #131527, #92730, #84595, #10575, #103874, #186102, #100031, #53174, #187152, #102491, #148891, #61448, #55170, #175946, #155536, #143932, #153225, #8299, #160955, #184287, #126740, #95794, #127349, #151085, #154838, #198527, #162289, #124239, #9199, #81451, #30281, #138196, #108474 ) ) ;
#101451=AXIS2_PLACEMENT_3D ( 'NONE', #37820, #193511, #103496 ) ;
#101455=ORIENTED_EDGE ( 'NONE', *, *, #196650, .F. ) ;
#101463=CARTESIAN_POINT ( 'NONE',  ( 5.000000000000000888, -130.0000000000000000, -13.99999999999999822 ) ) ;
#101594=ORIENTED_EDGE ( 'NONE', *, *, #3260, .F. ) ;
#101661=ORIENTED_EDGE ( 'NONE', *, *, #60782, .T. ) ;
#101690=DIRECTION ( 'NONE',  ( -5.392603844284257652E-33, -1.000000000000000000, -0.000000000000000000 ) ) ;
#101839=EDGE_CURVE ( 'NONE', #94667, #33072, #193790, .T. ) ;
#101956=EDGE_CURVE ( 'NONE', #161389, #166994, #74330, .T. ) ;
#102009=CARTESIAN_POINT ( 'NONE',  ( -193.3062444957834884, -155.7167183371838064, -15.00000000000000000 ) ) ;
#102080=AXIS2_PLACEMENT_3D ( 'NONE', #183308, #14442, #28648 ) ;
#102233=AXIS2_PLACEMENT_3D ( 'NONE', #131583, #86075, #7224 ) ;
#102359=EDGE_CURVE ( 'NONE', #169284, #125859, #86823, .T. ) ;
#102491=ADVANCED_FACE ( 'NONE', ( #70667 ), #12010, .F. ) ;
#102499=EDGE_LOOP ( 'NONE', ( #156107, #123289, #129157, #57917, #119440 ) ) ;
#102515=EDGE_CURVE ( 'NONE', #178033, #197949, #122646, .T. ) ;
#102575=FILL_AREA_STYLE ('',( #42899 ) ) ;
#102745=ORIENTED_EDGE ( 'NONE', *, *, #70632, .F. ) ;
#102754=CIRCLE ( 'NONE', #199602, 59.99999999999998579 ) ;
#102933=CARTESIAN_POINT ( 'NONE',  ( -193.3062444957834884, -155.7167183371838064, 0.000000000000000000 ) ) ;
#102945=ORIENTED_EDGE ( 'NONE', *, *, #157036, .F. ) ;
#102961=CARTESIAN_POINT ( 'NONE',  ( -11.30153831258470731, -180.0000000000000000, -15.00000000000000000 ) ) ;
#102989=DIRECTION ( 'NONE',  ( 0.000000000000000000, 0.000000000000000000, -1.000000000000000000 ) ) ;
#103058=CARTESIAN_POINT ( 'NONE',  ( -9.141470119588789092E-16, -69.45486021086043138, -12.99263613531267936 ) ) ;
#103239=EDGE_CURVE ( 'NONE', #94667, #174040, #133572, .T. ) ;
#103328=ORIENTED_EDGE ( 'NONE', *, *, #27433, .F. ) ;
#103446=ORIENTED_EDGE ( 'NONE', *, *, #111919, .T. ) ;
#103464=CARTESIAN_POINT ( 'NONE',  ( -5.000000000000000000, -120.0000000000000142, 0.0009999999999992653654 ) ) ;
#103496=DIRECTION ( 'NONE',  ( 1.000000000000000000, 5.372046893347532792E-15, 0.000000000000000000 ) ) ;
#103517=CYLINDRICAL_SURFACE ( 'NONE', #60587, 214.0437394197456911 ) ;
#103750=ORIENTED_EDGE ( 'NONE', *, *, #72556, .F. ) ;
#103874=ADVANCED_FACE ( 'NONE', ( #145221 ), #178582, .T. ) ;
#103939=DIRECTION ( 'NONE',  ( 0.000000000000000000, 0.000000000000000000, -1.000000000000000000 ) ) ;
#103948=ORIENTED_EDGE ( 'NONE', *, *, #79148, .T. ) ;
#104325=CARTESIAN_POINT ( 'NONE',  ( -11.30153831258470731, -180.0000000000000000, 1.787262988391354872E-28 ) ) ;
#104413=EDGE_LOOP ( 'NONE', ( #186853, #23912, #140170, #52275, #200108 ) ) ;
#104487=AXIS2_PLACEMENT_3D ( 'NONE', #29111, #134301, #91731 ) ;
#104558=DIRECTION ( 'NONE',  ( -1.000000000000000000, -6.451865313697283898E-33, -1.908195823574487804E-15 ) ) ;
#104576=DIRECTION ( 'NONE',  ( -0.000000000000000000, -0.000000000000000000, 1.000000000000000000 ) ) ;
#104637=AXIS2_PLACEMENT_3D ( 'NONE', #61936, #30626, #47791 ) ;
#104667=ORIENTED_EDGE ( 'NONE', *, *, #87523, .F. ) ;
#104835=EDGE_LOOP ( 'NONE', ( #93430, #77881, #44969, #175881 ) ) ;
#104851=VECTOR ( 'NONE', #198064, 1000.000000000000000 ) ;
#104911=FACE_OUTER_BOUND ( 'NONE', #177110, .T. ) ;
#104927=LINE ( 'NONE', #151440, #76671 ) ;
#105034=VECTOR ( 'NONE', #158617, 1000.000000000000000 ) ;
#105109=CARTESIAN_POINT ( 'NONE',  ( 11.30153831258471797, -180.0000000000000000, -4.999999999999994671 ) ) ;
#105243=ADVANCED_FACE ( 'NONE', ( #80374 ), #197544, .F. ) ;
#105397=ORIENTED_EDGE ( 'NONE', *, *, #32795, .F. ) ;
#105428=DIRECTION ( 'NONE',  ( -1.000000000000000000, 0.000000000000000000, 0.000000000000000000 ) ) ;
#105455=EDGE_LOOP ( 'NONE', ( #163204, #52043, #68684, #167702 ) ) ;
#105513=EDGE_LOOP ( 'NONE', ( #54205, #126304, #46297, #38658, #160920, #120854 ) ) ;
#105526=CARTESIAN_POINT ( 'NONE',  ( -11.30153831258471975, -180.0000000000000000, -4.999999999999999112 ) ) ;
#105697=ORIENTED_EDGE ( 'NONE', *, *, #48243, .T. ) ;
#105984=CARTESIAN_POINT ( 'NONE',  ( 193.3062444957835453, -155.7167183371837496, -4.999999999999999112 ) ) ;
#105998=CARTESIAN_POINT ( 'NONE',  ( -2.649999999999999911, -165.0000000000000000, -15.00000000000000000 ) ) ;
#105999=ORIENTED_EDGE ( 'NONE', *, *, #50678, .T. ) ;
#106027=CARTESIAN_POINT ( 'NONE',  ( -11.30153831258471975, -180.0000000000000000, -4.999999999999999112 ) ) ;
#106066=CARTESIAN_POINT ( 'NONE',  ( -193.3062444957834884, -155.7167183371838064, 0.000000000000000000 ) ) ;
#106224=DIRECTION ( 'NONE',  ( -1.000000000000000000, 0.000000000000000000, 0.000000000000000000 ) ) ;
#106289=EDGE_LOOP ( 'NONE', ( #150748, #69993, #119880, #87663 ) ) ;
#106368=EDGE_CURVE ( 'NONE', #19466, #14496, #69040, .T. ) ;
#106405=CARTESIAN_POINT ( 'NONE',  ( -11.30153831258470731, -188.0000000000000000, -4.999999999999999112 ) ) ;
#106509=DIRECTION ( 'NONE',  ( -1.000000000000000000, 0.000000000000000000, -5.421010862427521184E-16 ) ) ;
#106542=EDGE_CURVE ( 'NONE', #197949, #64290, #56212, .T. ) ;
#106884=CARTESIAN_POINT ( 'NONE',  ( 7.992609269207028790E-30, -165.0000000000000000, -15.00000000000000000 ) ) ;
#106902=CARTESIAN_POINT ( 'NONE',  ( 2.082452769671597245E-15, -69.45644693201178654, -14.99410988519313470 ) ) ;
#106992=DIRECTION ( 'NONE',  ( 0.000000000000000000, 0.000000000000000000, -1.000000000000000000 ) ) ;
#107014=SPHERICAL_SURFACE ( 'NONE', #124254, 10.00000000000000000 ) ;
#107041=ORIENTED_EDGE ( 'NONE', *, *, #140339, .T. ) ;
#107057=CARTESIAN_POINT ( 'NONE',  ( 19.78966525663867060, -34.76164524278549095, -6.188629846543125979 ) ) ;
#107115=FACE_OUTER_BOUND ( 'NONE', #4394, .T. ) ;
#107179=DIRECTION ( 'NONE',  ( -0.000000000000000000, -0.000000000000000000, 1.000000000000000000 ) ) ;
#107181=CARTESIAN_POINT ( 'NONE',  ( -3.573655867282028392E-15, 2.428612866367529932E-14, 1.984260520772446048E-44 ) ) ;
#107221=LINE ( 'NONE', #31395, #131463 ) ;
#107239=LINE ( 'NONE', #168910, #76488 ) ;
#107282=CARTESIAN_POINT ( 'NONE',  ( -4.622231866529366047E-30, -105.0000000000000000, -15.00000000000000000 ) ) ;
#107369=EDGE_LOOP ( 'NONE', ( #12478, #117942, #98630, #70139 ) ) ;
#107406=DIRECTION ( 'NONE',  ( 5.392603844284257652E-33, -1.000000000000000000, 0.000000000000000000 ) ) ;
#107568=EDGE_CURVE ( 'NONE', #150536, #141411, #109916, .T. ) ;
#107732=CARTESIAN_POINT ( 'NONE',  ( 9.656827144875922642, -71.74905178543389184, -4.999999999999999112 ) ) ;
#107806=AXIS2_PLACEMENT_3D ( 'NONE', #121394, #44569, #106224 ) ;
#107837=ORIENTED_EDGE ( 'NONE', *, *, #221, .T. ) ;
#108125=ORIENTED_EDGE ( 'NONE', *, *, #53169, .T. ) ;
#108199=TOROIDAL_SURFACE ( 'NONE', #98512, 206.0437394197456342, 8.000000000000000000 ) ;
#108359=VECTOR ( 'NONE', #90265, 1000.000000000000000 ) ;
#108474=ADVANCED_FACE ( 'NONE', ( #133905 ), #42893, .F. ) ;
#108521=( NAMED_UNIT ( * ) PLANE_ANGLE_UNIT ( ) SI_UNIT ( $, .RADIAN. ) );
#108639=CARTESIAN_POINT ( 'NONE',  ( -69.65682714487590488, -71.74905178543390605, -4.999999999999999112 ) ) ;
#108855=VECTOR ( 'NONE', #77384, 1000.000000000000000 ) ;
#108955=EDGE_CURVE ( 'NONE', #142920, #96037, #113913, .T. ) ;
#109002=AXIS2_PLACEMENT_3D ( 'NONE', #17532, #62026, #123691 ) ;
#109252=VECTOR ( 'NONE', #198768, 1000.000000000000000 ) ;
#109345=CARTESIAN_POINT ( 'NONE',  ( -6.856101608890825108E-16, -71.74905178543389184, -12.99263613531267936 ) ) ;
#109364=ORIENTED_EDGE ( 'NONE', *, *, #119692, .F. ) ;
#109628=VECTOR ( 'NONE', #199556, 1000.000000000000000 ) ;
#109638=DIRECTION ( 'NONE',  ( 0.000000000000000000, 0.000000000000000000, -1.000000000000000000 ) ) ;
#109759=DIRECTION ( 'NONE',  ( 0.000000000000000000, -1.000000000000000000, 0.000000000000000000 ) ) ;
#109916=B_SPLINE_CURVE_WITH_KNOTS ( 'NONE', 3,
 ( #168691, #179926, #41393, #197076, #183881, #103058, #121199 ),
 .UNSPECIFIED., .F., .F.,
 ( 4, 3, 4 ),
 ( -4.032110379226884939E-05, 0.000000000000000000, 0.006882574723720362095 ),
 .UNSPECIFIED. ) ;
#109939=CARTESIAN_POINT ( 'NONE',  ( -3.573655867282028392E-15, 2.428612866367529932E-14, -15.00000000000000000 ) ) ;
#110017=APPLICATION_CONTEXT ( 'automotive_design' ) ;
#110171=DIRECTION ( 'NONE',  ( -1.000000000000000000, -1.070572202317115416E-14, 0.000000000000000000 ) ) ;
#110184=DIRECTION ( 'NONE',  ( -1.000000000000000000, 5.392603844284257652E-33, 0.000000000000000000 ) ) ;
#110500=DIRECTION ( 'NONE',  ( 1.000000000000000000, 0.000000000000000000, 0.000000000000000000 ) ) ;
#110722=VECTOR ( 'NONE', #99709, 1000.000000000000000 ) ;
#110877=CARTESIAN_POINT ( 'NONE',  ( -27.86473085795038429, -129.0000000000000000, -13.99999999999999822 ) ) ;
#110895=ORIENTED_EDGE ( 'NONE', *, *, #54327, .T. ) ;
#110908=DIRECTION ( 'NONE',  ( 1.000000000000000000, 0.000000000000000000, 0.000000000000000000 ) ) ;
#110945=CARTESIAN_POINT ( 'NONE',  ( 5.000000000000000888, -130.0000000000000000, -13.99999999999999822 ) ) ;
#111163=CARTESIAN_POINT ( 'NONE',  ( -27.53954565730104065, -29.01074954818684404, -5.289573041754675131 ) ) ;
#111356=ORIENTED_EDGE ( 'NONE', *, *, #38347, .F. ) ;
#111368=CARTESIAN_POINT ( 'NONE',  ( -5.000000000000000888, -130.0000000000000000, -13.99999999999999822 ) ) ;
#111475=CARTESIAN_POINT ( 'NONE',  ( -3.573655867282028392E-15, 2.428612866367529932E-14, 1.984260520772446048E-44 ) ) ;
#111591=ORIENTED_EDGE ( 'NONE', *, *, #84711, .F. ) ;
#111792=CARTESIAN_POINT ( 'NONE',  ( 18.25458402832055071, -35.60444695113565672, -12.00144453093060903 ) ) ;
#111919=EDGE_CURVE ( 'NONE', #74166, #59417, #62256, .T. ) ;
#111936=CARTESIAN_POINT ( 'NONE',  ( -9.656827144875922642, -71.74905178543390605, 8.936314941956774358E-29 ) ) ;
#111972=ORIENTED_EDGE ( 'NONE', *, *, #100961, .T. ) ;
#112165=CARTESIAN_POINT ( 'NONE',  ( -25.19092422046364987, -31.08406191321079959, -7.296300659524873389 ) ) ;
#112219=ORIENTED_EDGE ( 'NONE', *, *, #955, .T. ) ;
#112589=EDGE_LOOP ( 'NONE', ( #95298, #182725, #71984, #155588, #137832, #150184, #118355, #47328 ) ) ;
#112632=CARTESIAN_POINT ( 'NONE',  ( -10.31942656230733313, -38.65189766944586580, -12.74745618418806536 ) ) ;
#112877=DIRECTION ( 'NONE',  ( -0.1178549842436473205, -0.9930308165857339997, 6.133374237849950220E-17 ) ) ;
#112934=DIRECTION ( 'NONE',  ( 0.000000000000000000, 0.000000000000000000, -1.000000000000000000 ) ) ;
#112941=DIRECTION ( 'NONE',  ( 0.000000000000000000, 0.000000000000000000, -1.000000000000000000 ) ) ;
#113146=CARTESIAN_POINT ( 'NONE',  ( -18.25439838449807795, -35.60454171183379657, -12.00154358691121637 ) ) ;
#113156=CARTESIAN_POINT ( 'NONE',  ( 2.310831529832237923E-15, -71.74905152827281540, -14.99410988490250496 ) ) ;
#113182=SURFACE_SIDE_STYLE ('',( #67681 ) ) ;
#113277=EDGE_CURVE ( 'NONE', #142969, #33072, #10770, .T. ) ;
#113411=DIRECTION ( 'NONE',  ( 0.000000000000000000, 0.000000000000000000, 1.000000000000000000 ) ) ;
#113517=DIRECTION ( 'NONE',  ( 0.000000000000000000, 0.000000000000000000, -1.000000000000000000 ) ) ;
#113563=EDGE_LOOP ( 'NONE', ( #49544, #172759, #173515, #199403, #36160 ) ) ;
#113618=CARTESIAN_POINT ( 'NONE',  ( -12.85938658117095912, -37.87800364893588068, -12.00565553424693022 ) ) ;
#113764=CARTESIAN_POINT ( 'NONE',  ( 27.53984522711021299, -29.01046520254151773, -5.289306513719187031 ) ) ;
#113913=CIRCLE ( 'NONE', #117258, 10.00000000000000000 ) ;
#113933=ORIENTED_EDGE ( 'NONE', *, *, #94568, .F. ) ;
#114028=DIRECTION ( 'NONE',  ( 1.000000000000000000, 0.000000000000000000, 0.000000000000000000 ) ) ;
#114054=AXIS2_PLACEMENT_3D ( 'NONE', #140840, #79169, #110500 ) ;
#114169=PRESENTATION_STYLE_ASSIGNMENT (( #129339 ) ) ;
#114198=AXIS2_PLACEMENT_3D ( 'NONE', #84395, #6556, #69242 ) ;
#114244=DIRECTION ( 'NONE',  ( 0.000000000000000000, 0.000000000000000000, -1.000000000000000000 ) ) ;
#114384=EDGE_LOOP ( 'NONE', ( #30881, #123581, #23400, #31597 ) ) ;
#114410=ADVANCED_FACE ( 'NONE', ( #136877 ), #93340, .F. ) ;
#114737=CARTESIAN_POINT ( 'NONE',  ( 19.24578484527059175, -180.9428398739492820, -15.00000000000000000 ) ) ;
#114870=CARTESIAN_POINT ( 'NONE',  ( 2.649999999999999911, -165.0000000000000000, -15.00000000000000000 ) ) ;
#114874=AXIS2_PLACEMENT_3D ( 'NONE', #36756, #162116, #19615 ) ;
#115010=CARTESIAN_POINT ( 'NONE',  ( -27.86273085795037829, -28.69962071417356242, 0.000000000000000000 ) ) ;
#115029=CARTESIAN_POINT ( 'NONE',  ( 14.64477982082356533, -37.22763889967101392, -11.21824398509625986 ) ) ;
#115048=CARTESIAN_POINT ( 'NONE',  ( -19.99999999999998224, -188.0000000000000000, -4.999999999999999112 ) ) ;
#115065=CIRCLE ( 'NONE', #128038, 59.99999999999998579 ) ;
#115132=DIRECTION ( 'NONE',  ( 1.000000000000000000, 0.000000000000000000, 0.000000000000000000 ) ) ;
#115140=ORIENTED_EDGE ( 'NONE', *, *, #152109, .F. ) ;
#115163=CARTESIAN_POINT ( 'NONE',  ( -3.791881235938239776E-15, -78.65691688641813073, -15.00000000000000000 ) ) ;
#115175=DIRECTION ( 'NONE',  ( 0.000000000000000000, 0.000000000000000000, 1.000000000000000000 ) ) ;
#115303=CIRCLE ( 'NONE', #157160, 59.99999999999998579 ) ;
#115350=ORIENTED_EDGE ( 'NONE', *, *, #95040, .T. ) ;
#115461=CARTESIAN_POINT ( 'NONE',  ( -69.65682714487590488, -71.74905178543390605, -15.00000000000000000 ) ) ;
#115764=CIRCLE ( 'NONE', #44756, 2.649999999999999911 ) ;
#116009=VERTEX_POINT ( 'NONE', #71985 ) ;
#116028=DIRECTION ( 'NONE',  ( 0.000000000000000000, 0.000000000000000000, 1.000000000000000000 ) ) ;
#116118=ORIENTED_EDGE ( 'NONE', *, *, #74851, .T. ) ;
#116219=DIRECTION ( 'NONE',  ( -0.000000000000000000, -0.000000000000000000, 1.000000000000000000 ) ) ;
#116340=ORIENTED_EDGE ( 'NONE', *, *, #123873, .T. ) ;
#116584=ORIENTED_EDGE ( 'NONE', *, *, #68983, .F. ) ;
#116598=EDGE_CURVE ( 'NONE', #116009, #184761, #139899, .T. ) ;
#116739=DIRECTION ( 'NONE',  ( -0.000000000000000000, -0.000000000000000000, -1.000000000000000000 ) ) ;
#117189=ORIENTED_EDGE ( 'NONE', *, *, #164677, .F. ) ;
#117258=AXIS2_PLACEMENT_3D ( 'NONE', #181415, #104558, #51322 ) ;
#117425=CYLINDRICAL_SURFACE ( 'NONE', #173793, 59.99999999999998579 ) ;
#117487=CIRCLE ( 'NONE', #101451, 61.99999999999998579 ) ;
#117533=FACE_OUTER_BOUND ( 'NONE', #181148, .T. ) ;
#117546=AXIS2_PLACEMENT_3D ( 'NONE', #150091, #104576, #149096 ) ;
#117580=AXIS2_PLACEMENT_3D ( 'NONE', #42318, #60441, #89802 ) ;
#117635=CARTESIAN_POINT ( 'NONE',  ( -18.50634305796425849, -35.46236190392534837, -8.314214632502698876 ) ) ;
#117655=LINE ( 'NONE', #177348, #98876 ) ;
#117665=CIRCLE ( 'NONE', #75655, 214.0437394197456911 ) ;
#117754=VECTOR ( 'NONE', #171898, 1000.000000000000000 ) ;
#117942=ORIENTED_EDGE ( 'NONE', *, *, #106542, .T. ) ;
#118110=DIRECTION ( 'NONE',  ( -0.000000000000000000, -0.000000000000000000, 1.000000000000000000 ) ) ;
#118125=VERTEX_POINT ( 'NONE', #95759 ) ;
#118171=DIRECTION ( 'NONE',  ( -5.392603844284257652E-33, -1.000000000000000000, -0.000000000000000000 ) ) ;
#118198=EDGE_CURVE ( 'NONE', #160176, #166994, #154945, .T. ) ;
#118200=DIRECTION ( 'NONE',  ( 1.000000000000000000, -4.336808689942018352E-17, 0.000000000000000000 ) ) ;
#118257=CIRCLE ( 'NONE', #163433, 61.99999999999998579 ) ;
#118355=ORIENTED_EDGE ( 'NONE', *, *, #59958, .F. ) ;
#118409=AXIS2_PLACEMENT_3D ( 'NONE', #187072, #65678, #155705 ) ;
#118444=ORIENTED_EDGE ( 'NONE', *, *, #166889, .T. ) ;
#118510=DIRECTION ( 'NONE',  ( -0.000000000000000000, -0.000000000000000000, 1.000000000000000000 ) ) ;
#118688=FACE_OUTER_BOUND ( 'NONE', #181883, .T. ) ;
#118717=DIRECTION ( 'NONE',  ( 1.000000000000000000, -4.336808689942017120E-17, 0.000000000000000000 ) ) ;
#118743=CARTESIAN_POINT ( 'NONE',  ( -4.622231866529366047E-30, -105.0000000000000000, -15.00000000000000000 ) ) ;
#118785=VERTEX_POINT ( 'NONE', #19915 ) ;
#118962=CIRCLE ( 'NONE', #31768, 10.00000000000000000 ) ;
#118963=EDGE_CURVE ( 'NONE', #169284, #49756, #97668, .T. ) ;
#118990=EDGE_CURVE ( 'NONE', #139926, #167341, #16889, .T. ) ;
#119403=CARTESIAN_POINT ( 'NONE',  ( 22.73749492396215288, -155.7167183371838064, -4.999999999999999112 ) ) ;
#119440=ORIENTED_EDGE ( 'NONE', *, *, #50976, .F. ) ;
#119505=DIRECTION ( 'NONE',  ( -1.000000000000000000, 0.000000000000000000, 0.000000000000000000 ) ) ;
#119624=DIRECTION ( 'NONE',  ( 0.9526137857479310966, -0.3041824702427718408, 0.000000000000000000 ) ) ;
#119692=EDGE_CURVE ( 'NONE', #141411, #101229, #74305, .T. ) ;
#119783=CARTESIAN_POINT ( 'NONE',  ( -69.65682714487590488, -71.74905178543390605, -4.999999999999999112 ) ) ;
#119836=ORIENTED_EDGE ( 'NONE', *, *, #196650, .T. ) ;
#119880=ORIENTED_EDGE ( 'NONE', *, *, #164988, .F. ) ;
#120095=DIRECTION ( 'NONE',  ( -1.000000000000000000, 0.000000000000000000, 0.000000000000000000 ) ) ;
#120150=DIRECTION ( 'NONE',  ( -1.000000000000000000, 5.392603844284257652E-33, 0.000000000000000000 ) ) ;
#120204=FACE_OUTER_BOUND ( 'NONE', #69262, .T. ) ;
#120467=EDGE_LOOP ( 'NONE', ( #124062, #112219, #159076, #67375 ) ) ;
#120473=CYLINDRICAL_SURFACE ( 'NONE', #93454, 2.649999999999999911 ) ;
#120589=CARTESIAN_POINT ( 'NONE',  ( 193.3062444957835453, -155.7167183371837496, -4.999999999999999112 ) ) ;
#120801=CIRCLE ( 'NONE', #65939, 8.000000000000007105 ) ;
#120854=ORIENTED_EDGE ( 'NONE', *, *, #160051, .F. ) ;
#120942=AXIS2_PLACEMENT_3D ( 'NONE', #151040, #138819, #93301 ) ;
#121047=B_SPLINE_CURVE_WITH_KNOTS ( 'NONE', 3,
 ( #109345, #171027, #32518, #94170, #155849, #79002, #187216 ),
 .UNSPECIFIED., .F., .F.,
 ( 4, 3, 4 ),
 ( 0.006882574723720362095, 0.01376514944744072419, 0.01380547055123299352 ),
 .UNSPECIFIED. ) ;
#121085=CIRCLE ( 'NONE', #153416, 2.649999999999999911 ) ;
#121199=CARTESIAN_POINT ( 'NONE',  ( -6.856101608890825108E-16, -71.74905178543389184, -12.99263613531267936 ) ) ;
#121322=CARTESIAN_POINT ( 'NONE',  ( 11.30153831258471797, -180.0000000000000000, -4.999999999999999112 ) ) ;
#121394=CARTESIAN_POINT ( 'NONE',  ( -4.718528363748727840E-30, -105.0000000000000000, -13.00000000000000000 ) ) ;
#121465=EDGE_CURVE ( 'NONE', #151273, #66675, #25821, .T. ) ;
#121547=FACE_OUTER_BOUND ( 'NONE', #123851, .T. ) ;
#121589=FACE_OUTER_BOUND ( 'NONE', #47384, .T. ) ;
#121599=CARTESIAN_POINT ( 'NONE',  ( -19.88080942482812929, -34.70959879495532618, -5.862652211910081235 ) ) ;
#121697=CIRCLE ( 'NONE', #34532, 59.99999999999998579 ) ;
#121702=( NAMED_UNIT ( * ) SI_UNIT ( $, .STERADIAN. ) SOLID_ANGLE_UNIT ( ) );
#122355=FACE_OUTER_BOUND ( 'NONE', #155112, .T. ) ;
#122541=VERTEX_POINT ( 'NONE', #89281 ) ;
#122577=ADVANCED_FACE ( 'NONE', ( #151946 ), #167673, .F. ) ;
#122613=CARTESIAN_POINT ( 'NONE',  ( -69.65682714487590488, -71.74905178543390605, -4.999999999999999112 ) ) ;
#122646=CIRCLE ( 'NONE', #87155, 216.0437394197456342 ) ;
#122782=ORIENTED_EDGE ( 'NONE', *, *, #154620, .F. ) ;
#122815=CARTESIAN_POINT ( 'NONE',  ( -2.649999999999999911, -105.0000000000000000, -13.00000000000000000 ) ) ;
#122895=CARTESIAN_POINT ( 'NONE',  ( 2.649999999999999911, -165.0000000000000000, -15.00000000000000000 ) ) ;
#123091=CARTESIAN_POINT ( 'NONE',  ( -69.65682714487590488, -71.74905178543390605, -4.999999999999999112 ) ) ;
#123141=DIRECTION ( 'NONE',  ( 1.000000000000000000, 0.000000000000000000, 0.000000000000000000 ) ) ;
#123289=ORIENTED_EDGE ( 'NONE', *, *, #152109, .T. ) ;
#123581=ORIENTED_EDGE ( 'NONE', *, *, #118963, .T. ) ;
#123595=CARTESIAN_POINT ( 'NONE',  ( -21.23184647844206197, -181.1785498424364675, 1.787262988391354872E-28 ) ) ;
#123691=DIRECTION ( 'NONE',  ( -1.000000000000000000, 0.000000000000000000, 0.000000000000000000 ) ) ;
#123851=EDGE_LOOP ( 'NONE', ( #69843, #4872, #57827, #156696, #18602 ) ) ;
#123873=EDGE_CURVE ( 'NONE', #188447, #38864, #93309, .T. ) ;
#123877=ORIENTED_EDGE ( 'NONE', *, *, #74851, .F. ) ;
#123916=DIRECTION ( 'NONE',  ( -0.000000000000000000, -0.000000000000000000, -1.000000000000000000 ) ) ;
#124049=CARTESIAN_POINT ( 'NONE',  ( 1.667840370490710761E-14, -64.85621347262014069, -14.99999966871768642 ) ) ;
#124062=ORIENTED_EDGE ( 'NONE', *, *, #64134, .T. ) ;
#124070=EDGE_CURVE ( 'NONE', #142350, #74166, #96625, .T. ) ;
#124117=ORIENTED_EDGE ( 'NONE', *, *, #84711, .T. ) ;
#124214=LINE ( 'NONE', #155557, #156386 ) ;
#124239=ADVANCED_FACE ( 'NONE', ( #83028 ), #188244, .F. ) ;
#124254=AXIS2_PLACEMENT_3D ( 'NONE', #106027, #134400, #151554 ) ;
#124538=EDGE_LOOP ( 'NONE', ( #194519, #185331, #103750, #87247, #147224, #13989 ) ) ;
#124807=DIRECTION ( 'NONE',  ( -1.000000000000000000, 0.000000000000000000, 0.000000000000000000 ) ) ;
#124933=CARTESIAN_POINT ( 'NONE',  ( -11.30153831258470731, -190.0000000000000000, -15.00000000000000000 ) ) ;
#125047=DIRECTION ( 'NONE',  ( -1.000000000000000000, 0.000000000000000000, 0.000000000000000000 ) ) ;
#125065=CARTESIAN_POINT ( 'NONE',  ( 2.310831529832237923E-15, -71.74905152827281540, -14.99410988490250496 ) ) ;
#125228=PLANE ( 'NONE',  #58020 ) ;
#125256=ORIENTED_EDGE ( 'NONE', *, *, #50192, .F. ) ;
#125293=CARTESIAN_POINT ( 'NONE',  ( -193.3062444957834884, -155.7167183371838064, -4.999999999999999112 ) ) ;
#125541=CARTESIAN_POINT ( 'NONE',  ( 7.652493125987820832, -39.26116846142902261, -13.00000000000000000 ) ) ;
#125701=CARTESIAN_POINT ( 'NONE',  ( 69.65682714487590488, -71.74905178543389184, -13.00000000000000000 ) ) ;
#125859=VERTEX_POINT ( 'NONE', #138504 ) ;
#125887=CARTESIAN_POINT ( 'NONE',  ( -21.23184647844206197, -181.1785498424364675, -15.00000000000000000 ) ) ;
#125957=ORIENTED_EDGE ( 'NONE', *, *, #150678, .T. ) ;
#126084=DIRECTION ( 'NONE',  ( -0.000000000000000000, -0.000000000000000000, -1.000000000000000000 ) ) ;
#126215=FACE_BOUND ( 'NONE', #105513, .T. ) ;
#126304=ORIENTED_EDGE ( 'NONE', *, *, #157314, .F. ) ;
#126572=CARTESIAN_POINT ( 'NONE',  ( -19.99999999999998224, -188.0000000000000000, 0.000000000000000000 ) ) ;
#126598=ORIENTED_EDGE ( 'NONE', *, *, #82917, .T. ) ;
#126740=ADVANCED_FACE ( 'NONE', ( #25148 ), #73639, .F. ) ;
#126812=B_SPLINE_CURVE_WITH_KNOTS ( 'NONE', 3,
 ( #35320, #19169, #6959, #80818, #143478, #128310, #146475, #64671, #67643, #97956, #113146, #51484, #127316, #158655, #112165, #23152, #52474, #68639, #142496, #111163, #130295, #188030 ),
 .UNSPECIFIED., .F., .F.,
 ( 4, 2, 2, 2, 2, 2, 2, 2, 2, 2, 4 ),
 ( 0.008245893658555575323, 0.01147022081997697146, 0.01308238440068766953, 0.01469454798139836760, 0.01791887514281974986, 0.02114320230424113906, 0.02759185662708390011, 0.03081618378850527543, 0.03242834736921596656, 0.03323442915957131039, 0.03404051094992665422 ),
 .UNSPECIFIED. ) ;
#126945=CARTESIAN_POINT ( 'NONE',  ( 26.55164451606355769, -29.92006817138308605, -6.154309889040165515 ) ) ;
#127044=CYLINDRICAL_SURFACE ( 'NONE', #82498, 2.649999999999999911 ) ;
#127193=FACE_BOUND ( 'NONE', #132838, .T. ) ;
#127316=CARTESIAN_POINT ( 'NONE',  ( -22.30831786103663816, -33.25057925659813662, -9.512335543930488413 ) ) ;
#127349=ADVANCED_FACE ( 'NONE', ( #147325 ), #158119, .F. ) ;
#127492=CARTESIAN_POINT ( 'NONE',  ( -11.30153831258470731, -180.0000000000000000, 1.787262988391354872E-28 ) ) ;
#127511=VERTEX_POINT ( 'NONE', #80409 ) ;
#127534=AXIS2_PLACEMENT_3D ( 'NONE', #11861, #136175, #197850 ) ;
#127795=CARTESIAN_POINT ( 'NONE',  ( -8.334442550624215684, -39.12824798328761489, -13.00000000000136957 ) ) ;
#127883=AXIS2_PLACEMENT_3D ( 'NONE', #105526, #185344, #106509 ) ;
#127977=ORIENTED_EDGE ( 'NONE', *, *, #82288, .F. ) ;
#127999=EDGE_CURVE ( 'NONE', #116009, #193478, #163252, .T. ) ;
#128038=AXIS2_PLACEMENT_3D ( 'NONE', #122613, #91257, #198479 ) ;
#128280=ORIENTED_EDGE ( 'NONE', *, *, #92125, .T. ) ;
#128310=CARTESIAN_POINT ( 'NONE',  ( -12.73180063597635403, -37.92326222289558757, -14.26362963886643875 ) ) ;
#128323=CARTESIAN_POINT ( 'NONE',  ( 2.995967610389833449E-15, -76.33425854457907178, -14.99989890116611768 ) ) ;
#128725=EDGE_CURVE ( 'NONE', #164433, #96037, #76196, .T. ) ;
#128786=CARTESIAN_POINT ( 'NONE',  ( -11.92151346184467897, -38.18361175107895633, -12.32871365052710999 ) ) ;
#128801=DIRECTION ( 'NONE',  ( -0.000000000000000000, -0.000000000000000000, -1.000000000000000000 ) ) ;
#128894=EDGE_CURVE ( 'NONE', #43824, #155176, #180442, .T. ) ;
#128919=EDGE_LOOP ( 'NONE', ( #999, #103328, #46184, #182554 ) ) ;
#129015=DIRECTION ( 'NONE',  ( 1.000000000000000000, 0.000000000000000000, 0.000000000000000000 ) ) ;
#129071=CARTESIAN_POINT ( 'NONE',  ( -69.65682714487590488, -71.74905178543390605, -15.00000000000000000 ) ) ;
#129083=DIRECTION ( 'NONE',  ( 0.000000000000000000, -1.000000000000000000, 0.000000000000000000 ) ) ;
#129087=CARTESIAN_POINT ( 'NONE',  ( 7.992609269207028790E-30, -165.0000000000000000, -15.00000000000000000 ) ) ;
#129157=ORIENTED_EDGE ( 'NONE', *, *, #63651, .T. ) ;
#129216=ORIENTED_EDGE ( 'NONE', *, *, #62612, .T. ) ;
#129339=SURFACE_STYLE_USAGE ( .BOTH. , #113182 ) ;
#129370=CARTESIAN_POINT ( 'NONE',  ( 11.30153831258470731, -188.0000000000000000, -15.00000000000000000 ) ) ;
#129575=ORIENTED_EDGE ( 'NONE', *, *, #43624, .F. ) ;
#130085=LINE ( 'NONE', #51280, #195156 ) ;
#130179=AXIS2_PLACEMENT_3D ( 'NONE', #115461, #37611, #193308 ) ;
#130283=CARTESIAN_POINT ( 'NONE',  ( -10.59477242850411649, -90.60836494048552936, 0.000000000000000000 ) ) ;
#130295=CARTESIAN_POINT ( 'NONE',  ( -27.70075874562641616, -28.85686966938180475, -5.145719711754212611 ) ) ;
#130358=EDGE_CURVE ( 'NONE', #70507, #182160, #161307, .T. ) ;
#130486=ADVANCED_FACE ( 'NONE', ( #29479 ), #120473, .F. ) ;
#130599=CIRCLE ( 'NONE', #182456, 40.00000000000002132 ) ;
#130897=DIRECTION ( 'NONE',  ( -0.000000000000000000, -0.000000000000000000, 1.000000000000000000 ) ) ;
#130939=CARTESIAN_POINT ( 'NONE',  ( -7.656827144875921753, -71.74905178543390605, -4.999999999999999112 ) ) ;
#130978=ORIENTED_EDGE ( 'NONE', *, *, #4625, .F. ) ;
#131222=AXIS2_PLACEMENT_3D ( 'NONE', #41329, #102989, #89815 ) ;
#131281=EDGE_LOOP ( 'NONE', ( #95856, #195692, #44066, #22869 ) ) ;
#131284=CARTESIAN_POINT ( 'NONE',  ( -12.73749492396214578, -155.7167183371837496, -13.00000000000000000 ) ) ;
#131326=CARTESIAN_POINT ( 'NONE',  ( -69.65682714487590488, -71.74905178543390605, -15.00000000000000000 ) ) ;
#131360=ORIENTED_EDGE ( 'NONE', *, *, #60782, .F. ) ;
#131463=VECTOR ( 'NONE', #49543, 1000.000000000000000 ) ;
#131510=ORIENTED_EDGE ( 'NONE', *, *, #199827, .T. ) ;
#131527=ADVANCED_FACE ( 'NONE', ( #198974 ), #138289, .F. ) ;
#131583=CARTESIAN_POINT ( 'NONE',  ( -193.3062444957834884, -155.7167183371838064, -15.00000000000000000 ) ) ;
#131638=VECTOR ( 'NONE', #199198, 1000.000000000000000 ) ;
#131941=ORIENTED_EDGE ( 'NONE', *, *, #57594, .T. ) ;
#131991=ORIENTED_EDGE ( 'NONE', *, *, #121465, .F. ) ;
#132148=CARTESIAN_POINT ( 'NONE',  ( -69.65682714487590488, -71.74905178543390605, -4.999999999999999112 ) ) ;
#132163=EDGE_CURVE ( 'NONE', #132746, #142969, #185860, .T. ) ;
#132273=DIRECTION ( 'NONE',  ( -1.000000000000000000, 0.000000000000000000, 0.000000000000000000 ) ) ;
#132278=CARTESIAN_POINT ( 'NONE',  ( 7.992609269207028790E-30, -165.0000000000000000, -15.00000000000000000 ) ) ;
#132284=ORIENTED_EDGE ( 'NONE', *, *, #143733, .F. ) ;
#132311=ORIENTED_EDGE ( 'NONE', *, *, #140339, .F. ) ;
#132369=ORIENTED_EDGE ( 'NONE', *, *, #52560, .F. ) ;
#132390=DIRECTION ( 'NONE',  ( 1.000000000000000000, 0.000000000000000000, 0.000000000000000000 ) ) ;
#132407=EDGE_CURVE ( 'NONE', #171657, #65708, #98186, .T. ) ;
#132462=CARTESIAN_POINT ( 'NONE',  ( -69.65682714487590488, -71.74905178543390605, 8.936314941956774358E-29 ) ) ;
#132746=VERTEX_POINT ( 'NONE', #68699 ) ;
#132800=CARTESIAN_POINT ( 'NONE',  ( -19.11512514549023578, -35.13775691452683247, -7.538968404279507318 ) ) ;
#132838=EDGE_LOOP ( 'NONE', ( #131991, #131360 ) ) ;
#132987=VERTEX_POINT ( 'NONE', #71707 ) ;
#133353=FACE_OUTER_BOUND ( 'NONE', #158864, .T. ) ;
#133361=VERTEX_POINT ( 'NONE', #179913 ) ;
#133568=VERTEX_POINT ( 'NONE', #149549 ) ;
#133572=CIRCLE ( 'NONE', #81856, 10.00000000000000000 ) ;
#133619=DIRECTION ( 'NONE',  ( 0.000000000000000000, 0.000000000000000000, 1.000000000000000000 ) ) ;
#133655=VECTOR ( 'NONE', #101002, 1000.000000000000000 ) ;
#133691=PLANE ( 'NONE',  #150704 ) ;
#133746=ORIENTED_EDGE ( 'NONE', *, *, #132163, .T. ) ;
#133845=EDGE_LOOP ( 'NONE', ( #135751, #74080, #183067, #28587 ) ) ;
#133905=FACE_OUTER_BOUND ( 'NONE', #11242, .T. ) ;
#134024=CARTESIAN_POINT ( 'NONE',  ( -193.3062444957834884, -155.7167183371838064, -15.00000000000000000 ) ) ;
#134053=AXIS2_PLACEMENT_3D ( 'NONE', #191766, #99750, #38095 ) ;
#134078=PRODUCT_DEFINITION_FORMATION_WITH_SPECIFIED_SOURCE ( 'ANY', '', #14587, .NOT_KNOWN. ) ;
#134144=VECTOR ( 'NONE', #96410, 1000.000000000000000 ) ;
#134189=ORIENTED_EDGE ( 'NONE', *, *, #69472, .F. ) ;
#134285=AXIS2_PLACEMENT_3D ( 'NONE', #40697, #23533, #54861 ) ;
#134301=DIRECTION ( 'NONE',  ( -0.000000000000000000, -0.000000000000000000, 1.000000000000000000 ) ) ;
#134357=FACE_OUTER_BOUND ( 'NONE', #107369, .T. ) ;
#134400=DIRECTION ( 'NONE',  ( -3.720488476448336339E-46, 1.000000000000000000, 7.149051953565418611E-31 ) ) ;
#134818=CARTESIAN_POINT ( 'NONE',  ( -19.29520783494825409, -35.03893545922181119, -7.263628290518377106 ) ) ;
#134853=EDGE_LOOP ( 'NONE', ( #123877, #26379, #54912, #125957 ) ) ;
#135206=EDGE_CURVE ( 'NONE', #160176, #161389, #56235, .T. ) ;
#135280=DIRECTION ( 'NONE',  ( -1.000000000000000000, 0.000000000000000000, 0.000000000000000000 ) ) ;
#135288=DIRECTION ( 'NONE',  ( -0.000000000000000000, -0.000000000000000000, 1.000000000000000000 ) ) ;
#135343=DIRECTION ( 'NONE',  ( 0.000000000000000000, 0.000000000000000000, -1.000000000000000000 ) ) ;
#135413=CARTESIAN_POINT ( 'NONE',  ( 19.97888994334924817, -34.65319547504296338, -7.500000000000000000 ) ) ;
#135608=ORIENTED_EDGE ( 'NONE', *, *, #53169, .F. ) ;
#135627=FACE_OUTER_BOUND ( 'NONE', #104835, .T. ) ;
#135751=ORIENTED_EDGE ( 'NONE', *, *, #142962, .F. ) ;
#135807=CIRCLE ( 'NONE', #16283, 10.00000000000000000 ) ;
#135844=ORIENTED_EDGE ( 'NONE', *, *, #64962, .F. ) ;
#136175=DIRECTION ( 'NONE',  ( 1.000000000000000000, -4.336808689942017120E-17, 0.000000000000000000 ) ) ;
#136334=CARTESIAN_POINT ( 'NONE',  ( 22.73749492396215288, -155.7167183371838064, -15.00000000000000000 ) ) ;
#136346=LINE ( 'NONE', #105998, #18609 ) ;
#136877=FACE_OUTER_BOUND ( 'NONE', #14624, .T. ) ;
#137361=DIRECTION ( 'NONE',  ( -1.000000000000000000, 0.000000000000000000, 0.000000000000000000 ) ) ;
#137434=ORIENTED_EDGE ( 'NONE', *, *, #47812, .F. ) ;
#137566=VERTEX_POINT ( 'NONE', #81729 ) ;
#137595=CARTESIAN_POINT ( 'NONE',  ( 11.30153831258470731, -188.0000000000000000, -1.787262988391354872E-28 ) ) ;
#137756=CARTESIAN_POINT ( 'NONE',  ( -19.99999999999998224, -190.0000000000000000, -15.00000000000000000 ) ) ;
#137832=ORIENTED_EDGE ( 'NONE', *, *, #113277, .F. ) ;
#138051=ORIENTED_EDGE ( 'NONE', *, *, #135206, .F. ) ;
#138196=ADVANCED_FACE ( 'NONE', ( #104911 ), #199907, .F. ) ;
#138259=ORIENTED_EDGE ( 'NONE', *, *, #5261, .T. ) ;
#138289=CYLINDRICAL_SURFACE ( 'NONE', #117580, 59.99999999999998579 ) ;
#138504=CARTESIAN_POINT ( 'NONE',  ( 5.000000000000000888, -130.0000000000000000, -12.99999999999999822 ) ) ;
#138529=CARTESIAN_POINT ( 'NONE',  ( -3.573655867282025236E-15, -180.0000000000000000, -13.00000000000000000 ) ) ;
#138661=CARTESIAN_POINT ( 'NONE',  ( -20.73749492396214933, -155.7167183371837496, -4.999999999999999112 ) ) ;
#138819=DIRECTION ( 'NONE',  ( 0.000000000000000000, 0.000000000000000000, -1.000000000000000000 ) ) ;
#138820=ORIENTED_EDGE ( 'NONE', *, *, #79148, .F. ) ;
#138833=FACE_OUTER_BOUND ( 'NONE', #32389, .T. ) ;
#139232=CARTESIAN_POINT ( 'NONE',  ( 9.310586156219267749E-15, -64.87124026077280803, -14.99999901254159873 ) ) ;
#139302=LINE ( 'NONE', #136334, #42917 ) ;
#139548=EDGE_CURVE ( 'NONE', #97924, #142920, #75703, .T. ) ;
#139856=VECTOR ( 'NONE', #140753, 1000.000000000000000 ) ;
#139899=CIRCLE ( 'NONE', #156076, 214.0437394197456342 ) ;
#139926=VERTEX_POINT ( 'NONE', #75726 ) ;
#139973=DIRECTION ( 'NONE',  ( 0.000000000000000000, 0.000000000000000000, -1.000000000000000000 ) ) ;
#140170=ORIENTED_EDGE ( 'NONE', *, *, #102515, .F. ) ;
#140215=CARTESIAN_POINT ( 'NONE',  ( 5.000000000000000888, -140.0000000000000000, 0.0009999999999992653654 ) ) ;
#140219=CARTESIAN_POINT ( 'NONE',  ( 1.348150961071065097E-30, -64.82615989628266107, -15.00000000000000000 ) ) ;
#140278=DIRECTION ( 'NONE',  ( -1.000000000000000000, 0.000000000000000000, 0.000000000000000000 ) ) ;
#140290=DIRECTION ( 'NONE',  ( 1.000000000000000000, 0.000000000000000000, 0.000000000000000000 ) ) ;
#140294=CARTESIAN_POINT ( 'NONE',  ( -4.999999999999999112, -140.0000000000000000, 0.0009999999999992653654 ) ) ;
#140339=EDGE_CURVE ( 'NONE', #158522, #182127, #124214, .T. ) ;
#140753=DIRECTION ( 'NONE',  ( 4.336808689942017120E-17, 1.000000000000000000, 0.000000000000000000 ) ) ;
#140791=VECTOR ( 'NONE', #123916, 1000.000000000000000 ) ;
#140840=CARTESIAN_POINT ( 'NONE',  ( -193.3062444957834884, -155.7167183371838064, -15.00000000000000000 ) ) ;
#140861=DIRECTION ( 'NONE',  ( -0.000000000000000000, -0.000000000000000000, 1.000000000000000000 ) ) ;
#141041=AXIS2_PLACEMENT_3D ( 'NONE', #163691, #52497, #70680 ) ;
#141253=LINE ( 'NONE', #187784, #31615 ) ;
#141411=VERTEX_POINT ( 'NONE', #24026 ) ;
#141695=LINE ( 'NONE', #3186, #188985 ) ;
#142122=CARTESIAN_POINT ( 'NONE',  ( 25.19119763768592790, -31.08384082485095590, -7.296079031154174110 ) ) ;
#142266=FACE_OUTER_BOUND ( 'NONE', #198492, .T. ) ;
#142290=CARTESIAN_POINT ( 'NONE',  ( 193.3062444957835453, -155.7167183371837496, 0.000000000000000000 ) ) ;
#142350=VERTEX_POINT ( 'NONE', #49280 ) ;
#142457=CARTESIAN_POINT ( 'NONE',  ( 11.30153831258469843, -180.0000000000000000, -15.00000000000000000 ) ) ;
#142496=CARTESIAN_POINT ( 'NONE',  ( -27.21294631871472802, -29.31732793098551682, -5.578473613576554690 ) ) ;
#142519=CARTESIAN_POINT ( 'NONE',  ( -11.30153831258472508, -180.0000000000000000, -4.999999999999999112 ) ) ;
#142552=EDGE_LOOP ( 'NONE', ( #56279, #21060, #183485 ) ) ;
#142739=DIRECTION ( 'NONE',  ( 1.000000000000000000, -5.392603844284257652E-33, 0.000000000000000000 ) ) ;
#142748=ORIENTED_EDGE ( 'NONE', *, *, #71161, .T. ) ;
#142789=EDGE_CURVE ( 'NONE', #118785, #125859, #159860, .T. ) ;
#142920=VERTEX_POINT ( 'NONE', #142457 ) ;
#142962=EDGE_CURVE ( 'NONE', #142350, #184761, #175793, .T. ) ;
#142969=VERTEX_POINT ( 'NONE', #83757 ) ;
#142977=DIRECTION ( 'NONE',  ( -1.000000000000000000, 0.000000000000000000, 0.000000000000000000 ) ) ;
#143324=EDGE_CURVE ( 'NONE', #142920, #178033, #79163, .T. ) ;
#143478=CARTESIAN_POINT ( 'NONE',  ( -11.73768782171584313, -38.24263654170160720, -14.51834023846848254 ) ) ;
#143489=DIRECTION ( 'NONE',  ( -0.000000000000000000, -0.000000000000000000, 1.000000000000000000 ) ) ;
#143549=COLOUR_RGB ( '', 0.66274510, 0.83137255, 0.94901961) ;
#143654=DIRECTION ( 'NONE',  ( -1.000000000000000000, 0.000000000000000000, 0.000000000000000000 ) ) ;
#143667=VECTOR ( 'NONE', #43910, 1000.000000000000000 ) ;
#143705=CARTESIAN_POINT ( 'NONE',  ( 5.000000000000000888, -140.0000000000000000, 0.0009999999999992653654 ) ) ;
#143733=EDGE_CURVE ( 'NONE', #145279, #6627, #195401, .T. ) ;
#143754=PLANE ( 'NONE',  #57612 ) ;
#143786=ORIENTED_EDGE ( 'NONE', *, *, #50192, .T. ) ;
#143863=FACE_OUTER_BOUND ( 'NONE', #104413, .T. ) ;
#143932=ADVANCED_FACE ( 'NONE', ( #193969, #58428, #59409, #11953 ), #9945, .F. ) ;
#143946=EDGE_CURVE ( 'NONE', #150536, #127511, #92002, .T. ) ;
#144068=CARTESIAN_POINT ( 'NONE',  ( -27.86273085795036408, -28.69962071417357663, -15.00000000000000000 ) ) ;
#144211=DIRECTION ( 'NONE',  ( 0.000000000000000000, 0.000000000000000000, -1.000000000000000000 ) ) ;
#144348=CIRCLE ( 'NONE', #141041, 59.99999999999998579 ) ;
#144359=CARTESIAN_POINT ( 'NONE',  ( 12.23969591940464952, -38.08276121122112556, -12.22614352002200100 ) ) ;
#144376=CARTESIAN_POINT ( 'NONE',  ( 193.3062444957835453, -155.7167183371837496, -4.999999999999999112 ) ) ;
#144752=DIRECTION ( 'NONE',  ( 1.000000000000000000, 0.000000000000000000, 0.000000000000000000 ) ) ;
#144876=ADVANCED_FACE ( 'NONE', ( #171577 ), #153414, .T. ) ;
#144978=AXIS2_PLACEMENT_3D ( 'NONE', #102961, #148477, #115132 ) ;
#145221=FACE_OUTER_BOUND ( 'NONE', #20388, .T. ) ;
#145279=VERTEX_POINT ( 'NONE', #114870 ) ;
#145704=DIRECTION ( 'NONE',  ( 0.000000000000000000, 0.000000000000000000, -1.000000000000000000 ) ) ;
#145721=EDGE_LOOP ( 'NONE', ( #103446, #78109, #107837, #153502, #15374 ) ) ;
#145743=CYLINDRICAL_SURFACE ( 'NONE', #102233, 214.0437394197456342 ) ;
#146103=DIRECTION ( 'NONE',  ( -1.000000000000000000, 0.000000000000000000, 0.000000000000000000 ) ) ;
#146245=DIRECTION ( 'NONE',  ( 0.000000000000000000, 0.000000000000000000, 1.000000000000000000 ) ) ;
#146371=DIRECTION ( 'NONE',  ( 1.000000000000000000, -5.392603844284257652E-33, 0.000000000000000000 ) ) ;
#146432=CARTESIAN_POINT ( 'NONE',  ( 20.73749492396215288, -155.7167183371838064, -15.00000000000000000 ) ) ;
#146475=CARTESIAN_POINT ( 'NONE',  ( -13.21949426486139423, -37.75586497602908764, -14.12003558585129426 ) ) ;
#146484=CARTESIAN_POINT ( 'NONE',  ( -4.814824860968089633E-30, -78.67194367458512261, -15.00000000000000000 ) ) ;
#146774=AXIS2_PLACEMENT_3D ( 'NONE', #142290, #3770, #123141 ) ;
#147008=DIRECTION ( 'NONE',  ( -1.000000000000000000, 0.000000000000000000, 0.000000000000000000 ) ) ;
#147177=EDGE_LOOP ( 'NONE', ( #101161, #149118, #68925, #165354 ) ) ;
#147224=ORIENTED_EDGE ( 'NONE', *, *, #123873, .F. ) ;
#147325=FACE_OUTER_BOUND ( 'NONE', #79645, .T. ) ;
#147371=CARTESIAN_POINT ( 'NONE',  ( 12.86046501205820825, -37.87763584681607654, -12.00524328043752575 ) ) ;
#147449=DIRECTION ( 'NONE',  ( 4.336808689942018352E-17, -1.000000000000000000, 0.000000000000000000 ) ) ;
#147875=CARTESIAN_POINT ( 'NONE',  ( -4.999999999999999112, -140.0000000000000000, 0.0009999999999992653654 ) ) ;
#147958=VERTEX_POINT ( 'NONE', #2374 ) ;
#148291=CARTESIAN_POINT ( 'NONE',  ( -12.73749492396214578, -155.7167183371837496, -4.999999999999999112 ) ) ;
#148455=EDGE_CURVE ( 'NONE', #147958, #150223, #17946, .T. ) ;
#148477=DIRECTION ( 'NONE',  ( 0.000000000000000000, 0.000000000000000000, 1.000000000000000000 ) ) ;
#148692=ORIENTED_EDGE ( 'NONE', *, *, #108955, .F. ) ;
#148891=ADVANCED_FACE ( 'NONE', ( #117533 ), #67029, .T. ) ;
#149026=LINE ( 'NONE', #41850, #170435 ) ;
#149096=DIRECTION ( 'NONE',  ( -1.000000000000000000, 0.000000000000000000, 0.000000000000000000 ) ) ;
#149107=LINE ( 'NONE', #57099, #143667 ) ;
#149118=ORIENTED_EDGE ( 'NONE', *, *, #34170, .T. ) ;
#149144=AXIS2_PLACEMENT_3D ( 'NONE', #47587, #18248, #95065 ) ;
#149173=VERTEX_POINT ( 'NONE', #183194 ) ;
#149445=CARTESIAN_POINT ( 'NONE',  ( -69.65682714487590488, -71.74905178543390605, -13.00000000000000000 ) ) ;
#149535=EDGE_LOOP ( 'NONE', ( #109364, #115350, #92809, #174650, #189502 ) ) ;
#149549=CARTESIAN_POINT ( 'NONE',  ( -21.23184647844206552, -181.1785498424364675, -4.999999999999999112 ) ) ;
#149956=DIRECTION ( 'NONE',  ( -0.3041824702427711191, -0.9526137857479313187, 0.000000000000000000 ) ) ;
#149971=CARTESIAN_POINT ( 'NONE',  ( -19.52983155694575501, -34.90836132267833847, -6.822515721995922711 ) ) ;
#149973=CIRCLE ( 'NONE', #146774, 216.0437394197456911 ) ;
#150019=DIRECTION ( 'NONE',  ( 1.000000000000000000, 0.000000000000000000, 0.000000000000000000 ) ) ;
#150081=TOROIDAL_SURFACE ( 'NONE', #175900, 206.0437394197456911, 10.00000000000000000 ) ;
#150091=CARTESIAN_POINT ( 'NONE',  ( -193.3062444957834884, -155.7167183371838064, -4.999999999999999112 ) ) ;
#150184=ORIENTED_EDGE ( 'NONE', *, *, #199827, .F. ) ;
#150223=VERTEX_POINT ( 'NONE', #79976 ) ;
#150512=DIRECTION ( 'NONE',  ( 4.336808689942017120E-17, 1.000000000000000000, 0.000000000000000000 ) ) ;
#150536=VERTEX_POINT ( 'NONE', #16324 ) ;
#150553=DIRECTION ( 'NONE',  ( -1.000000000000000000, 0.000000000000000000, 0.000000000000000000 ) ) ;
#150678=EDGE_CURVE ( 'NONE', #118125, #22637, #118257, .T. ) ;
#150704=AXIS2_PLACEMENT_3D ( 'NONE', #147875, #71026, #179221 ) ;
#150748=ORIENTED_EDGE ( 'NONE', *, *, #25084, .T. ) ;
#150830=VECTOR ( 'NONE', #101123, 1000.000000000000000 ) ;
#150925=DIRECTION ( 'NONE',  ( -1.000000000000000000, 0.000000000000000000, 0.000000000000000000 ) ) ;
#151032=CIRCLE ( 'NONE', #28369, 69.99999999999998579 ) ;
#151040=CARTESIAN_POINT ( 'NONE',  ( 69.65682714487590488, -71.74905178543389184, 0.000000000000000000 ) ) ;
#151053=SPHERICAL_SURFACE ( 'NONE', #127883, 8.000000000000000000 ) ;
#151085=ADVANCED_FACE ( 'NONE', ( #89364 ), #151053, .F. ) ;
#151167=VERTEX_POINT ( 'NONE', #90345 ) ;
#151204=CARTESIAN_POINT ( 'NONE',  ( -10.59477242850411649, -90.60836494048552936, -4.999999999999999112 ) ) ;
#151273=VERTEX_POINT ( 'NONE', #45839 ) ;
#151275=ORIENTED_EDGE ( 'NONE', *, *, #142962, .T. ) ;
#151292=DIRECTION ( 'NONE',  ( 0.000000000000000000, 0.000000000000000000, -1.000000000000000000 ) ) ;
#151408=ADVANCED_FACE ( 'NONE', ( #138833 ), #46835, .F. ) ;
#151440=CARTESIAN_POINT ( 'NONE',  ( -4.999999999999999112, -140.0000000000000000, -13.00000000000000000 ) ) ;
#151543=CARTESIAN_POINT ( 'NONE',  ( -69.65682714487590488, -71.74905178543390605, 8.936314941956774358E-29 ) ) ;
#151554=DIRECTION ( 'NONE',  ( -1.000000000000000000, 0.000000000000000000, -5.204170427930421283E-16 ) ) ;
#151653=VECTOR ( 'NONE', #116739, 1000.000000000000000 ) ;
#151779=CYLINDRICAL_SURFACE ( 'NONE', #182265, 216.0437394197456342 ) ;
#151814=AXIS2_PLACEMENT_3D ( 'NONE', #78941, #5076, #114244 ) ;
#151864=EDGE_CURVE ( 'NONE', #147958, #178033, #7454, .T. ) ;
#151946=FACE_OUTER_BOUND ( 'NONE', #89567, .T. ) ;
#152109=EDGE_CURVE ( 'NONE', #64290, #174040, #169910, .T. ) ;
#152271=CARTESIAN_POINT ( 'NONE',  ( -3.573655867282028392E-15, 2.428612866367529932E-14, -15.00000000000000000 ) ) ;
#152540=LINE ( 'NONE', #135413, #104851 ) ;
#152778=EDGE_CURVE ( 'NONE', #99125, #118785, #53570, .T. ) ;
#152884=ORIENTED_EDGE ( 'NONE', *, *, #92125, .F. ) ;
#153035=CARTESIAN_POINT ( 'NONE',  ( -19.99999999999998224, -190.0000000000000000, -4.999999999999999112 ) ) ;
#153039=AXIS2_PLACEMENT_3D ( 'NONE', #9541, #118717, #24717 ) ;
#153225=ADVANCED_FACE ( 'NONE', ( #46776 ), #96981, .F. ) ;
#153236=LINE ( 'NONE', #122895, #109252 ) ;
#153414=CYLINDRICAL_SURFACE ( 'NONE', #43693, 216.0437394197456911 ) ;
#153416=AXIS2_PLACEMENT_3D ( 'NONE', #5434, #37781, #187511 ) ;
#153495=DIRECTION ( 'NONE',  ( 0.000000000000000000, 0.000000000000000000, -1.000000000000000000 ) ) ;
#153502=ORIENTED_EDGE ( 'NONE', *, *, #182203, .T. ) ;
#153598=AXIS2_PLACEMENT_3D ( 'NONE', #179231, #51860, #193385 ) ;
#153696=TOROIDAL_SURFACE ( 'NONE', #40705, 206.0437394197456911, 10.00000000000000000 ) ;
#153741=AXIS2_PLACEMENT_3D ( 'NONE', #111475, #171171, #66959 ) ;
#153933=CARTESIAN_POINT ( 'NONE',  ( -27.86273085795037474, -28.69962071417356242, -4.999999999999999112 ) ) ;
#153998=TOROIDAL_SURFACE ( 'NONE', #37365, 69.99999999999998579, 8.000000000000000000 ) ;
#154283=CARTESIAN_POINT ( 'NONE',  ( -5.000000000000000888, -130.0000000000000000, -13.99999999999999822 ) ) ;
#154502=ORIENTED_EDGE ( 'NONE', *, *, #85978, .F. ) ;
#154566=CARTESIAN_POINT ( 'NONE',  ( -3.573655867282028392E-15, 2.428612866367529932E-14, -15.00000000000000000 ) ) ;
#154620=EDGE_CURVE ( 'NONE', #36346, #41468, #85907, .T. ) ;
#154768=EDGE_CURVE ( 'NONE', #23117, #65708, #69890, .T. ) ;
#154838=ADVANCED_FACE ( 'NONE', ( #142266 ), #44072, .F. ) ;
#154945=CIRCLE ( 'NONE', #16115, 40.00000000000002132 ) ;
#155112=EDGE_LOOP ( 'NONE', ( #96287, #156731, #190441, #74605, #34302, #13167, #101455, #135608, #74322, #105397, #122782, #22345 ) ) ;
#155176=VERTEX_POINT ( 'NONE', #111936 ) ;
#155536=ADVANCED_FACE ( 'NONE', ( #177617 ), #158435, .T. ) ;
#155557=CARTESIAN_POINT ( 'NONE',  ( -19.99999999999998224, -190.0000000000000000, 0.000000000000000000 ) ) ;
#155560=CARTESIAN_POINT ( 'NONE',  ( 19.73275029929832414, -34.79402272588036737, -6.352102039474952555 ) ) ;
#155588=ORIENTED_EDGE ( 'NONE', *, *, #101839, .T. ) ;
#155691=ORIENTED_EDGE ( 'NONE', *, *, #30090, .F. ) ;
#155705=DIRECTION ( 'NONE',  ( -1.000000000000000000, 0.000000000000000000, 0.000000000000000000 ) ) ;
#155710=DIRECTION ( 'NONE',  ( -1.000000000000000000, -1.071875439572228152E-15, -5.204170427930421283E-16 ) ) ;
#155790=CARTESIAN_POINT ( 'NONE',  ( -22.73749492396214933, -155.7167183371837496, -4.999999999999999112 ) ) ;
#155849=CARTESIAN_POINT ( 'NONE',  ( -2.260530480648141910E-15, -78.64506293871966136, -12.99999966871702917 ) ) ;
#155865=ORIENTED_EDGE ( 'NONE', *, *, #65094, .F. ) ;
#155897=DIRECTION ( 'NONE',  ( 0.000000000000000000, 0.000000000000000000, -1.000000000000000000 ) ) ;
#155924=ORIENTED_EDGE ( 'NONE', *, *, #106368, .T. ) ;
#156076=AXIS2_PLACEMENT_3D ( 'NONE', #179189, #169957, #32446 ) ;
#156107=ORIENTED_EDGE ( 'NONE', *, *, #170373, .F. ) ;
#156386=VECTOR ( 'NONE', #17051, 1000.000000000000000 ) ;
#156399=CARTESIAN_POINT ( 'NONE',  ( 193.3062444957835453, -155.7167183371837496, -15.00000000000000000 ) ) ;
#156437=ADVANCED_FACE ( 'NONE', ( #121547 ), #195493, .F. ) ;
#156599=AXIS2_PLACEMENT_3D ( 'NONE', #227, #61895, #185260 ) ;
#156620=DIRECTION ( 'NONE',  ( -1.000000000000000000, 0.000000000000000000, 0.000000000000000000 ) ) ;
#156696=ORIENTED_EDGE ( 'NONE', *, *, #93154, .T. ) ;
#156731=ORIENTED_EDGE ( 'NONE', *, *, #118198, .T. ) ;
#156746=PRODUCT_DEFINITION_SHAPE ( 'NONE', 'NONE',  #52321 ) ;
#157036=EDGE_CURVE ( 'NONE', #40357, #57973, #31782, .T. ) ;
#157160=AXIS2_PLACEMENT_3D ( 'NONE', #119783, #40947, #146103 ) ;
#157307=CARTESIAN_POINT ( 'NONE',  ( 27.70335742114823319, -28.85434677204553111, -5.143381789178917529 ) ) ;
#157314=EDGE_CURVE ( 'NONE', #49756, #40748, #159077, .T. ) ;
#157452=DIRECTION ( 'NONE',  ( 0.000000000000000000, 0.000000000000000000, -1.000000000000000000 ) ) ;
#157478=VECTOR ( 'NONE', #181303, 1000.000000000000000 ) ;
#157727=LINE ( 'NONE', #80866, #117754 ) ;
#157737=EDGE_LOOP ( 'NONE', ( #174573, #116118, #42806, #86029 ) ) ;
#157903=DIRECTION ( 'NONE',  ( -1.000000000000000000, 0.000000000000000000, 0.000000000000000000 ) ) ;
#158119=TOROIDAL_SURFACE ( 'NONE', #54784, 69.99999999999998579, 8.000000000000000000 ) ;
#158181=CARTESIAN_POINT ( 'NONE',  ( -69.65682714487590488, -71.74905178543390605, 8.936314941956774358E-29 ) ) ;
#158204=CARTESIAN_POINT ( 'NONE',  ( -4.999999999999999112, -140.0000000000000000, -13.00000000000000000 ) ) ;
#158294=CARTESIAN_POINT ( 'NONE',  ( 14.65784320516234018, -37.23156113918972210, -13.64775320819145144 ) ) ;
#158355=B_SPLINE_CURVE_WITH_KNOTS ( 'NONE', 3,
 ( #4442, #127795, #20623, #112632, #5444, #128786, #190486, #113618, #175312, #87296, #41803, #12473, #167134, #164154, #55959, #28634, #9471, #117635, #11477, #132800, #134818, #149971, #179334, #181322, #90271, #121599, #29607, #183294, #73148, #198460 ),
 .UNSPECIFIED., .F., .F.,
 ( 4, 2, 2, 2, 2, 2, 2, 2, 2, 2, 2, 2, 2, 2, 4 ),
 ( 0.008686738875643574415, 0.01074815216733882375, 0.01280956545903407309, 0.01384027210488169776, 0.01487097875072932243, 0.01693239204242456830, 0.01899380533411981417, 0.02002451197996743537, 0.02105521862581505310, 0.02208592527166267083, 0.02311663191751028856, 0.02363198524043409743, 0.02414733856335790629, 0.02466269188628171516, 0.02517804520920552402 ),
 .UNSPECIFIED. ) ;
#158435=CYLINDRICAL_SURFACE ( 'NONE', #56634, 61.99999999999998579 ) ;
#158522=VERTEX_POINT ( 'NONE', #176272 ) ;
#158617=DIRECTION ( 'NONE',  ( 0.000000000000000000, 0.000000000000000000, 1.000000000000000000 ) ) ;
#158630=CARTESIAN_POINT ( 'NONE',  ( -5.000000000000000888, -130.0000000000000000, -15.00000000000000000 ) ) ;
#158655=CARTESIAN_POINT ( 'NONE',  ( -24.48769569731326357, -31.64124327689851768, -7.859335325863215260 ) ) ;
#158710=CARTESIAN_POINT ( 'NONE',  ( -19.24578484527059175, -180.9428398739492252, -4.999999999999999112 ) ) ;
#158864=EDGE_LOOP ( 'NONE', ( #75803, #128280, #10474, #6267, #14043, #36969 ) ) ;
#159076=ORIENTED_EDGE ( 'NONE', *, *, #57173, .T. ) ;
#159077=LINE ( 'NONE', #34751, #134144 ) ;
#159130=UNCERTAINTY_MEASURE_WITH_UNIT (LENGTH_MEASURE( 1.000000000000000082E-05 ), #82837, 'distance_accuracy_value', 'NONE');
#159210=VERTEX_POINT ( 'NONE', #125541 ) ;
#159563=PRODUCT_DEFINITION_CONTEXT ( 'detailed design', #60997, 'design' ) ;
#159726=COLOUR_RGB ( '', 0.66274510, 0.83137255, 0.94901961) ;
#159860=CIRCLE ( 'NONE', #134053, 1.000000000000000888 ) ;
#159900=CIRCLE ( 'NONE', #195451, 1.000000000000000888 ) ;
#160051=EDGE_CURVE ( 'NONE', #193517, #40598, #141695, .T. ) ;
#160176=VERTEX_POINT ( 'NONE', #163872 ) ;
#160287=CARTESIAN_POINT ( 'NONE',  ( 24.48796087919907905, -31.64103850882386126, -7.859127186814490074 ) ) ;
#160334=AXIS2_PLACEMENT_3D ( 'NONE', #105109, #168746, #28296 ) ;
#160535=CARTESIAN_POINT ( 'NONE',  ( 27.86273085795036408, -28.69962071417356242, -15.00000000000000000 ) ) ;
#160692=FILL_AREA_STYLE ('',( #191034 ) ) ;
#160920=ORIENTED_EDGE ( 'NONE', *, *, #57173, .F. ) ;
#160955=ADVANCED_FACE ( 'NONE', ( #161855 ), #88003, .F. ) ;
#161307=CIRCLE ( 'NONE', #61133, 8.000000000000000000 ) ;
#161389=VERTEX_POINT ( 'NONE', #40687 ) ;
#161855=FACE_OUTER_BOUND ( 'NONE', #75145, .T. ) ;
#161897=ORIENTED_EDGE ( 'NONE', *, *, #69568, .T. ) ;
#161919=EDGE_LOOP ( 'NONE', ( #182867, #116584, #155865, #86153, #49356, #168860 ) ) ;
#162116=DIRECTION ( 'NONE',  ( 0.000000000000000000, 0.000000000000000000, 1.000000000000000000 ) ) ;
#162283=CARTESIAN_POINT ( 'NONE',  ( 7.652493125987819944, -39.26116846142902261, -15.00000000000000000 ) ) ;
#162289=ADVANCED_FACE ( 'NONE', ( #86185 ), #133691, .F. ) ;
#162510=CARTESIAN_POINT ( 'NONE',  ( 5.000000000000000888, -140.0000000000000000, -15.00000000000000000 ) ) ;
#162766=AXIS2_PLACEMENT_3D ( 'NONE', #65384, #112877, #66381 ) ;
#162936=ORIENTED_EDGE ( 'NONE', *, *, #50976, .T. ) ;
#163179=ORIENTED_EDGE ( 'NONE', *, *, #71161, .F. ) ;
#163204=ORIENTED_EDGE ( 'NONE', *, *, #84050, .F. ) ;
#163252=LINE ( 'NONE', #114737, #151653 ) ;
#163282=ORIENTED_EDGE ( 'NONE', *, *, #69568, .F. ) ;
#163433=AXIS2_PLACEMENT_3D ( 'NONE', #132462, #54614, #85951 ) ;
#163532=VECTOR ( 'NONE', #146371, 1000.000000000000000 ) ;
#163663=B_SPLINE_CURVE_WITH_KNOTS ( 'NONE', 3,
 ( #15063, #185915, #188905, #107057, #155560, #76723, #169735, #186926, #92879, #16062, #1873, #77720, #63554, #48396, #84673, #115029, #5846, #81671, #147371, #144359, #98842, #20029, #23028, #22026, #176722, #99851 ),
 .UNSPECIFIED., .F., .F.,
 ( 4, 2, 2, 2, 2, 2, 2, 2, 2, 2, 2, 2, 4 ),
 ( 1.964780709336654224E-07, 0.001036009418421648520, 0.001553915888597004469, 0.002071822358772360418, 0.003107635299123065378, 0.004143448239473769036, 0.006215074120175169414, 0.008286700000876570660, 0.01035832588157797017, 0.01139413882192866732, 0.01242995176227936274, 0.01450157764298075705, 0.01657320352368214789 ),
 .UNSPECIFIED. ) ;
#163687=AXIS2_PLACEMENT_3D ( 'NONE', #125293, #40245, #178777 ) ;
#163691=CARTESIAN_POINT ( 'NONE',  ( 69.65682714487590488, -71.74905178543389184, -4.999999999999999112 ) ) ;
#163706=CYLINDRICAL_SURFACE ( 'NONE', #2569, 1.000000000000000888 ) ;
#163872=CARTESIAN_POINT ( 'NONE',  ( 7.652493125987819944, -39.26116846142902261, -15.00000000000000000 ) ) ;
#163926=ORIENTED_EDGE ( 'NONE', *, *, #78587, .T. ) ;
#163950=FACE_OUTER_BOUND ( 'NONE', #120467, .T. ) ;
#163970=EDGE_CURVE ( 'NONE', #193478, #188443, #199031, .T. ) ;
#164101=CARTESIAN_POINT ( 'NONE',  ( 69.65682714487590488, -71.74905178543389184, -4.999999999999999112 ) ) ;
#164154=CARTESIAN_POINT ( 'NONE',  ( -17.07994770534405760, -36.17121603258436835, -9.645916067152393580 ) ) ;
#164159=VERTEX_POINT ( 'NONE', #182952 ) ;
#164259=SURFACE_STYLE_FILL_AREA ( #102575 ) ;
#164368=AXIS2_PLACEMENT_3D ( 'NONE', #143705, #38544, #145704 ) ;
#164433=VERTEX_POINT ( 'NONE', #172748 ) ;
#164677=EDGE_CURVE ( 'NONE', #15380, #192038, #166718, .T. ) ;
#164690=CYLINDRICAL_SURFACE ( 'NONE', #183062, 216.0437394197456342 ) ;
#164722=CARTESIAN_POINT ( 'NONE',  ( 2.649999999999999911, -105.0000000000000000, -15.00000000000000000 ) ) ;
#164734=LINE ( 'NONE', #129370, #91909 ) ;
#164782=CARTESIAN_POINT ( 'NONE',  ( 19.97888994334922685, -34.65319547504297759, -5.000000000000000000 ) ) ;
#164886=AXIS2_PLACEMENT_3D ( 'NONE', #186511, #109638, #61143 ) ;
#164983=CARTESIAN_POINT ( 'NONE',  ( 11.30153831258470731, -180.0000000000000000, 0.000000000000000000 ) ) ;
#164988=EDGE_CURVE ( 'NONE', #171657, #188443, #53370, .T. ) ;
#165154=ORIENTED_EDGE ( 'NONE', *, *, #150678, .F. ) ;
#165193=CARTESIAN_POINT ( 'NONE',  ( 193.3062444957835453, -155.7167183371837496, -15.00000000000000000 ) ) ;
#165210=VERTEX_POINT ( 'NONE', #33887 ) ;
#165354=ORIENTED_EDGE ( 'NONE', *, *, #43996, .T. ) ;
#165999=CIRCLE ( 'NONE', #107806, 2.649999999999999911 ) ;
#166153=EDGE_CURVE ( 'NONE', #40748, #193517, #60740, .T. ) ;
#166248=EDGE_CURVE ( 'NONE', #133361, #132987, #107239, .T. ) ;
#166337=ORIENTED_EDGE ( 'NONE', *, *, #38962, .F. ) ;
#166377=FACE_OUTER_BOUND ( 'NONE', #105455, .T. ) ;
#166615=VECTOR ( 'NONE', #128801, 1000.000000000000000 ) ;
#166718=CIRCLE ( 'NONE', #95669, 214.0437394197456911 ) ;
#166772=DIRECTION ( 'NONE',  ( -1.000000000000000000, 0.000000000000000000, 0.000000000000000000 ) ) ;
#166889=EDGE_CURVE ( 'NONE', #74166, #137566, #177995, .T. ) ;
#166957=CARTESIAN_POINT ( 'NONE',  ( -4.999999999999999112, -140.0000000000000000, -15.00000000000000000 ) ) ;
#166994=VERTEX_POINT ( 'NONE', #70811 ) ;
#167081=DIRECTION ( 'NONE',  ( 0.000000000000000000, 0.000000000000000000, -1.000000000000000000 ) ) ;
#167124=DIRECTION ( 'NONE',  ( 0.000000000000000000, 0.000000000000000000, -1.000000000000000000 ) ) ;
#167128=LINE ( 'NONE', #103464, #108359 ) ;
#167134=CARTESIAN_POINT ( 'NONE',  ( -16.30299161242153971, -36.53133444124396334, -10.23071320450981680 ) ) ;
#167341=VERTEX_POINT ( 'NONE', #67851 ) ;
#167451=AXIS2_PLACEMENT_3D ( 'NONE', #176630, #180639, #55264 ) ;
#167452=PLANE ( 'NONE',  #1396 ) ;
#167673=TOROIDAL_SURFACE ( 'NONE', #48165, 206.0437394197456911, 8.000000000000000000 ) ;
#167678=CARTESIAN_POINT ( 'NONE',  ( 5.000000000000000888, -140.0000000000000000, -15.00000000000000000 ) ) ;
#167702=ORIENTED_EDGE ( 'NONE', *, *, #88386, .T. ) ;
#167704=AXIS2_PLACEMENT_3D ( 'NONE', #168786, #88982, #181020 ) ;
#167981=DIRECTION ( 'NONE',  ( -1.000000000000000000, 0.000000000000000000, 0.000000000000000000 ) ) ;
#167994=EDGE_CURVE ( 'NONE', #151167, #160176, #67962, .T. ) ;
#168100=PLANE ( 'NONE',  #33912 ) ;
#168389=ORIENTED_EDGE ( 'NONE', *, *, #65754, .T. ) ;
#168691=CARTESIAN_POINT ( 'NONE',  ( 1.251854463851703304E-30, -64.82615989628266107, -13.00000000000000000 ) ) ;
#168746=DIRECTION ( 'NONE',  ( -5.204170427930421283E-16, 0.000000000000000000, -1.000000000000000000 ) ) ;
#168786=CARTESIAN_POINT ( 'NONE',  ( -19.99999999999998224, -180.0000000000000000, -4.999999999999999112 ) ) ;
#168827=EDGE_CURVE ( 'NONE', #197193, #43824, #115303, .T. ) ;
#168852=DIRECTION ( 'NONE',  ( 0.000000000000000000, 0.000000000000000000, -1.000000000000000000 ) ) ;
#168860=ORIENTED_EDGE ( 'NONE', *, *, #102359, .F. ) ;
#168910=CARTESIAN_POINT ( 'NONE',  ( 5.000000000000001776, -120.0000000000000142, 0.0009999999999992653654 ) ) ;
#169095=VERTEX_POINT ( 'NONE', #130939 ) ;
#169228=AXIS2_PLACEMENT_3D ( 'NONE', #188027, #107179, #110171 ) ;
#169284=VERTEX_POINT ( 'NONE', #56107 ) ;
#169494=CIRCLE ( 'NONE', #66136, 10.00000000000000888 ) ;
#169735=CARTESIAN_POINT ( 'NONE',  ( 19.53216895467080860, -34.90705393983476768, -6.817813017276924015 ) ) ;
#169792=CARTESIAN_POINT ( 'NONE',  ( 69.65682714487590488, -71.74905178543389184, 0.000000000000000000 ) ) ;
#169903=ORIENTED_EDGE ( 'NONE', *, *, #166889, .F. ) ;
#169910=CIRCLE ( 'NONE', #195786, 59.99999999999998579 ) ;
#169926=ORIENTED_EDGE ( 'NONE', *, *, #170997, .T. ) ;
#169957=DIRECTION ( 'NONE',  ( -0.000000000000000000, -0.000000000000000000, 1.000000000000000000 ) ) ;
#170031=CARTESIAN_POINT ( 'NONE',  ( 2.310831529832237923E-15, -71.74905152827281540, -14.99410988490250496 ) ) ;
#170294=AXIS2_PLACEMENT_3D ( 'NONE', #63484, #106992, #199019 ) ;
#170373=EDGE_CURVE ( 'NONE', #64290, #30088, #107221, .T. ) ;
#170435=VECTOR ( 'NONE', #31, 1000.000000000000000 ) ;
#170464=AXIS2_PLACEMENT_3D ( 'NONE', #27145, #89789, #12963 ) ;
#170476=ORIENTED_EDGE ( 'NONE', *, *, #101839, .F. ) ;
#170648=DIRECTION ( 'NONE',  ( 0.000000000000000000, 0.000000000000000000, 1.000000000000000000 ) ) ;
#170649=ORIENTED_EDGE ( 'NONE', *, *, #154768, .F. ) ;
#170967=VECTOR ( 'NONE', #181424, 1000.000000000000000 ) ;
#170997=EDGE_CURVE ( 'NONE', #14496, #19466, #189649, .T. ) ;
#171027=CARTESIAN_POINT ( 'NONE',  ( -4.570733098192862111E-16, -74.04324336000735229, -12.99263613531267936 ) ) ;
#171074=CARTESIAN_POINT ( 'NONE',  ( 193.3062444957835453, -155.7167183371837496, -13.00000000000000000 ) ) ;
#171171=DIRECTION ( 'NONE',  ( 0.000000000000000000, 0.000000000000000000, -1.000000000000000000 ) ) ;
#171344=ORIENTED_EDGE ( 'NONE', *, *, #143324, .T. ) ;
#171397=CARTESIAN_POINT ( 'NONE',  ( 12.50000000000001066, -90.00000000000005684, -4.999999999999999112 ) ) ;
#171474=ORIENTED_EDGE ( 'NONE', *, *, #160051, .T. ) ;
#171571=DIRECTION ( 'NONE',  ( -1.000000000000000000, 0.000000000000000000, 0.000000000000000000 ) ) ;
#171577=FACE_OUTER_BOUND ( 'NONE', #23191, .T. ) ;
#171657=VERTEX_POINT ( 'NONE', #106405 ) ;
#171788=DIRECTION ( 'NONE',  ( -1.000000000000000000, 0.000000000000000000, 0.000000000000000000 ) ) ;
#171898=DIRECTION ( 'NONE',  ( 0.000000000000000000, 0.000000000000000000, -1.000000000000000000 ) ) ;
#171917=DIRECTION ( 'NONE',  ( 0.000000000000000000, 0.000000000000000000, 1.000000000000000000 ) ) ;
#172125=ORIENTED_EDGE ( 'NONE', *, *, #46506, .F. ) ;
#172430=CARTESIAN_POINT ( 'NONE',  ( -5.000000000000000888, -131.0000000000000000, -13.99999999999999822 ) ) ;
#172711=ORIENTED_EDGE ( 'NONE', *, *, #167994, .F. ) ;
#172718=AXIS2_PLACEMENT_3D ( 'NONE', #21105, #52434, #37267 ) ;
#172748=CARTESIAN_POINT ( 'NONE',  ( -11.30153831258470731, -190.0000000000000000, -4.999999999999999112 ) ) ;
#172759=ORIENTED_EDGE ( 'NONE', *, *, #64962, .T. ) ;
#172810=VECTOR ( 'NONE', #76282, 1000.000000000000000 ) ;
#172863=CARTESIAN_POINT ( 'NONE',  ( 7.656827144875921753, -71.74905178543389184, -4.999999999999999112 ) ) ;
#173389=DIRECTION ( 'NONE',  ( 0.000000000000000000, -1.000000000000000000, 0.000000000000000000 ) ) ;
#173480=CARTESIAN_POINT ( 'NONE',  ( 17.38119043544336506, -36.03980009027800691, -12.45558932256932039 ) ) ;
#173515=ORIENTED_EDGE ( 'NONE', *, *, #83344, .T. ) ;
#173550=DIRECTION ( 'NONE',  ( 0.000000000000000000, 0.000000000000000000, -1.000000000000000000 ) ) ;
#173596=DIRECTION ( 'NONE',  ( -1.000000000000000000, -4.336808689942018352E-17, 3.574525976782710619E-31 ) ) ;
#173793=AXIS2_PLACEMENT_3D ( 'NONE', #179123, #113411, #144752 ) ;
#173884=CARTESIAN_POINT ( 'NONE',  ( 11.30153831258470021, -180.0000000000000000, -4.999999999999999112 ) ) ;
#174039=ORIENTED_EDGE ( 'NONE', *, *, #43478, .T. ) ;
#174040=VERTEX_POINT ( 'NONE', #107732 ) ;
#174573=ORIENTED_EDGE ( 'NONE', *, *, #57594, .F. ) ;
#174650=ORIENTED_EDGE ( 'NONE', *, *, #111919, .F. ) ;
#174867=LINE ( 'NONE', #191029, #133655 ) ;
#175062=DIRECTION ( 'NONE',  ( 0.000000000000000000, 0.000000000000000000, -1.000000000000000000 ) ) ;
#175134=ORIENTED_EDGE ( 'NONE', *, *, #175799, .T. ) ;
#175312=CARTESIAN_POINT ( 'NONE',  ( -13.16448406242845159, -37.77297734889211966, -11.88662703519201180 ) ) ;
#175793=LINE ( 'NONE', #146432, #105034 ) ;
#175799=EDGE_CURVE ( 'NONE', #15380, #19836, #149026, .T. ) ;
#175872=( LENGTH_UNIT ( ) NAMED_UNIT ( * ) SI_UNIT ( .MILLI., .METRE. ) );
#175881=ORIENTED_EDGE ( 'NONE', *, *, #151864, .T. ) ;
#175896=CARTESIAN_POINT ( 'NONE',  ( 193.3062444957835453, -155.7167183371837496, -15.00000000000000000 ) ) ;
#175900=AXIS2_PLACEMENT_3D ( 'NONE', #88515, #60158, #197698 ) ;
#175909=AXIS2_PLACEMENT_3D ( 'NONE', #148291, #13755, #88604 ) ;
#175946=ADVANCED_FACE ( 'NONE', ( #118688 ), #103517, .F. ) ;
#175959=DIRECTION ( 'NONE',  ( -1.000000000000000000, 0.000000000000000000, 0.000000000000000000 ) ) ;
#176069=CARTESIAN_POINT ( 'NONE',  ( -11.30153831258470731, -180.0000000000000000, -4.999999999999999112 ) ) ;
#176272=CARTESIAN_POINT ( 'NONE',  ( -11.30153831258470731, -190.0000000000000000, 0.000000000000000000 ) ) ;
#176320=AXIS2_PLACEMENT_3D ( 'NONE', #186130, #179433, #77925 ) ;
#176353=ORIENTED_EDGE ( 'NONE', *, *, #152778, .F. ) ;
#176426=DIRECTION ( 'NONE',  ( 0.000000000000000000, 0.000000000000000000, 1.000000000000000000 ) ) ;
#176575=EDGE_LOOP ( 'NONE', ( #102745, #108125, #51152 ) ) ;
#176630=CARTESIAN_POINT ( 'NONE',  ( -69.65682714487590488, -71.74905178543390605, -4.999999999999999112 ) ) ;
#176645=ORIENTED_EDGE ( 'NONE', *, *, #97058, .T. ) ;
#176722=CARTESIAN_POINT ( 'NONE',  ( 8.334387768958743337, -39.12825866091939986, -13.00000000000000000 ) ) ;
#176759=ADVANCED_FACE ( 'NONE', ( #133353 ), #163706, .T. ) ;
#177110=EDGE_LOOP ( 'NONE', ( #154502, #199319, #8666, #21881 ) ) ;
#177115=AXIS2_PLACEMENT_3D ( 'NONE', #105984, #44325, #184817 ) ;
#177348=CARTESIAN_POINT ( 'NONE',  ( -19.97888994334924107, -34.65319547504297759, -7.500000000000000000 ) ) ;
#177550=DIRECTION ( 'NONE',  ( -0.000000000000000000, -0.000000000000000000, 1.000000000000000000 ) ) ;
#177588=CARTESIAN_POINT ( 'NONE',  ( 11.30153831258471797, -180.0000000000000000, -4.999999999999999112 ) ) ;
#177617=FACE_OUTER_BOUND ( 'NONE', #134853, .T. ) ;
#177807=ORIENTED_EDGE ( 'NONE', *, *, #130358, .F. ) ;
#177995=LINE ( 'NONE', #39462, #150830 ) ;
#178033=VERTEX_POINT ( 'NONE', #12035 ) ;
#178067=EDGE_CURVE ( 'NONE', #19466, #6627, #136346, .T. ) ;
#178304=EDGE_CURVE ( 'NONE', #22637, #19836, #183296, .T. ) ;
#178582=SPHERICAL_SURFACE ( 'NONE', #94873, 10.00000000000000000 ) ;
#178640=ORIENTED_EDGE ( 'NONE', *, *, #66709, .T. ) ;
#178777=DIRECTION ( 'NONE',  ( 1.000000000000000000, 0.000000000000000000, 0.000000000000000000 ) ) ;
#178854=DIRECTION ( 'NONE',  ( -1.000000000000000000, 1.246178594180516623E-14, 0.000000000000000000 ) ) ;
#178958=CIRCLE ( 'NONE', #162766, 8.000000000000000000 ) ;
#179109=STYLED_ITEM ( 'NONE', ( #90372 ), #7058 ) ;
#179123=CARTESIAN_POINT ( 'NONE',  ( 69.65682714487590488, -71.74905178543389184, -15.00000000000000000 ) ) ;
#179154=ORIENTED_EDGE ( 'NONE', *, *, #39357, .T. ) ;
#179189=CARTESIAN_POINT ( 'NONE',  ( -193.3062444957834884, -155.7167183371838064, 0.000000000000000000 ) ) ;
#179221=DIRECTION ( 'NONE',  ( 4.336808689942018352E-17, -1.000000000000000000, 0.000000000000000000 ) ) ;
#179231=CARTESIAN_POINT ( 'NONE',  ( 69.65682714487590488, -71.74905178543389184, -15.00000000000000000 ) ) ;
#179278=EDGE_LOOP ( 'NONE', ( #163926, #174039, #133746, #84136, #142748, #73738 ) ) ;
#179287=VECTOR ( 'NONE', #86791, 1000.000000000000000 ) ;
#179334=CARTESIAN_POINT ( 'NONE',  ( -19.60206085084869443, -34.86781819333700838, -6.670742825288880518 ) ) ;
#179433=DIRECTION ( 'NONE',  ( -0.3041824702427711746, 0.9526137857479314297, 1.533086186985162281E-15 ) ) ;
#179862=DIRECTION ( 'NONE',  ( 1.000000000000000000, 0.000000000000000000, 0.000000000000000000 ) ) ;
#179869=EDGE_CURVE ( 'NONE', #8593, #155176, #102754, .T. ) ;
#179913=CARTESIAN_POINT ( 'NONE',  ( 5.000000000000001776, -120.0000000000000142, -13.00000000000000000 ) ) ;
#179920=CARTESIAN_POINT ( 'NONE',  ( 69.65682714487590488, -71.74905178543389184, -4.999999999999999112 ) ) ;
#179926=CARTESIAN_POINT ( 'NONE',  ( -2.285367203649863287E-16, -64.83960026421343059, -13.00000000000000000 ) ) ;
#180200=DIRECTION ( 'NONE',  ( 0.000000000000000000, 0.000000000000000000, -1.000000000000000000 ) ) ;
#180442=LINE ( 'NONE', #92353, #109628 ) ;
#180586=CARTESIAN_POINT ( 'NONE',  ( -4.999999999999999112, -140.0000000000000000, 0.0009999999999992653654 ) ) ;
#180639=DIRECTION ( 'NONE',  ( -0.000000000000000000, -0.000000000000000000, -1.000000000000000000 ) ) ;
#180718=CIRCLE ( 'NONE', #22488, 61.99999999999998579 ) ;
#180808=EDGE_LOOP ( 'NONE', ( #85773, #16373, #186475, #166337 ) ) ;
#180858=CARTESIAN_POINT ( 'NONE',  ( 5.000000000000000888, -140.0000000000000000, -13.00000000000000000 ) ) ;
#181020=DIRECTION ( 'NONE',  ( 0.000000000000000000, 0.000000000000000000, -1.000000000000000000 ) ) ;
#181073=CARTESIAN_POINT ( 'NONE',  ( -19.24578484527059175, -180.9428398739491684, -15.00000000000000000 ) ) ;
#181144=DIRECTION ( 'NONE',  ( 1.000000000000000000, 0.000000000000000000, 0.000000000000000000 ) ) ;
#181148=EDGE_LOOP ( 'NONE', ( #176645, #3944, #86268, #172125, #118444 ) ) ;
#181303=DIRECTION ( 'NONE',  ( -4.336808689942017120E-17, -1.000000000000000000, 0.000000000000000000 ) ) ;
#181322=CARTESIAN_POINT ( 'NONE',  ( -19.73163076381609216, -34.79465882235955121, -6.355234051081566804 ) ) ;
#181415=CARTESIAN_POINT ( 'NONE',  ( 11.30153831258470731, -180.0000000000000000, -4.999999999999999112 ) ) ;
#181424=DIRECTION ( 'NONE',  ( 1.000000000000000000, -5.392603844284257652E-33, 0.000000000000000000 ) ) ;
#181565=ORIENTED_EDGE ( 'NONE', *, *, #221, .F. ) ;
#181659=DIRECTION ( 'NONE',  ( -1.000000000000000000, 0.000000000000000000, 0.000000000000000000 ) ) ;
#181883=EDGE_LOOP ( 'NONE', ( #175134, #56448, #87766, #132369, #117189 ) ) ;
#181894=CARTESIAN_POINT ( 'NONE',  ( -3.573655867281984216E-15, 2.428612866367529932E-14, -13.00000000000000000 ) ) ;
#181939=DIRECTION ( 'NONE',  ( 1.000000000000000000, -4.336808689942018352E-17, 0.000000000000000000 ) ) ;
#182127=VERTEX_POINT ( 'NONE', #17119 ) ;
#182160=VERTEX_POINT ( 'NONE', #78771 ) ;
#182203=EDGE_CURVE ( 'NONE', #193478, #142350, #186344, .T. ) ;
#182265=AXIS2_PLACEMENT_3D ( 'NONE', #74935, #133619, #181144 ) ;
#182284=DIRECTION ( 'NONE',  ( 0.000000000000000000, 0.000000000000000000, -1.000000000000000000 ) ) ;
#182456=AXIS2_PLACEMENT_3D ( 'NONE', #181894, #44370, #137361 ) ;
#182554=ORIENTED_EDGE ( 'NONE', *, *, #151864, .F. ) ;
#182725=ORIENTED_EDGE ( 'NONE', *, *, #101956, .F. ) ;
#182867=ORIENTED_EDGE ( 'NONE', *, *, #48487, .F. ) ;
#182914=AXIS2_PLACEMENT_3D ( 'NONE', #187808, #61449, #49277 ) ;
#182952=CARTESIAN_POINT ( 'NONE',  ( -11.30153831258471442, -180.0000000000000000, -15.00000000000000000 ) ) ;
#183062=AXIS2_PLACEMENT_3D ( 'NONE', #102009, #115175, #72682 ) ;
#183067=ORIENTED_EDGE ( 'NONE', *, *, #127999, .F. ) ;
#183194=CARTESIAN_POINT ( 'NONE',  ( -5.000000000000000000, -130.0000000000000000, -13.00000000000000000 ) ) ;
#183294=CARTESIAN_POINT ( 'NONE',  ( -19.96598992073551671, -34.66064120484043087, -5.351514793237743817 ) ) ;
#183296=CIRCLE ( 'NONE', #189784, 61.99999999999998579 ) ;
#183308=CARTESIAN_POINT ( 'NONE',  ( 11.30153831258470731, -180.0000000000000000, -15.00000000000000000 ) ) ;
#183482=ORIENTED_EDGE ( 'NONE', *, *, #63651, .F. ) ;
#183485=ORIENTED_EDGE ( 'NONE', *, *, #101956, .T. ) ;
#183867=AXIS2_PLACEMENT_3D ( 'NONE', #95927, #35254, #156620 ) ;
#183881=CARTESIAN_POINT ( 'NONE',  ( -6.856101608890819192E-16, -67.16067257189654072, -12.99988689144064402 ) ) ;
#183903=ORIENTED_EDGE ( 'NONE', *, *, #27433, .T. ) ;
#184009=VECTOR ( 'NONE', #150512, 1000.000000000000000 ) ;
#184104=DIRECTION ( 'NONE',  ( -4.336808689942018352E-17, 1.000000000000000000, 0.000000000000000000 ) ) ;
#184262=DIRECTION ( 'NONE',  ( 0.000000000000000000, 0.000000000000000000, 1.000000000000000000 ) ) ;
#184287=ADVANCED_FACE ( 'NONE', ( #65353 ), #153998, .F. ) ;
#184761=VERTEX_POINT ( 'NONE', #99672 ) ;
#184817=DIRECTION ( 'NONE',  ( -1.000000000000000000, 0.000000000000000000, 0.000000000000000000 ) ) ;
#185260=DIRECTION ( 'NONE',  ( -1.000000000000000000, 0.000000000000000000, 0.000000000000000000 ) ) ;
#185331=ORIENTED_EDGE ( 'NONE', *, *, #77828, .F. ) ;
#185344=DIRECTION ( 'NONE',  ( -3.875508829633682909E-46, 1.000000000000000000, 7.149051953565419487E-31 ) ) ;
#185608=CIRCLE ( 'NONE', #98395, 61.99999999999998579 ) ;
#185767=ADVANCED_FACE ( 'NONE', ( #32804 ), #28184, .T. ) ;
#185817=ORIENTED_EDGE ( 'NONE', *, *, #154620, .T. ) ;
#185860=CIRCLE ( 'NONE', #47004, 206.0437394197456911 ) ;
#185915=CARTESIAN_POINT ( 'NONE',  ( 19.97888994334925172, -34.65319547504297049, -5.351457953959465108 ) ) ;
#186001=VECTOR ( 'NONE', #176426, 1000.000000000000000 ) ;
#186102=ADVANCED_FACE ( 'NONE', ( #100435 ), #38779, .T. ) ;
#186130=CARTESIAN_POINT ( 'NONE',  ( 2.973862142520697471, -93.04182470242776049, -4.999999999999999112 ) ) ;
#186344=CIRCLE ( 'NONE', #163687, 214.0437394197456342 ) ;
#186475=ORIENTED_EDGE ( 'NONE', *, *, #179869, .F. ) ;
#186511=CARTESIAN_POINT ( 'NONE',  ( 193.3062444957835453, -155.7167183371837496, -13.00000000000000000 ) ) ;
#186762=DIRECTION ( 'NONE',  ( -0.000000000000000000, -0.000000000000000000, 1.000000000000000000 ) ) ;
#186853=ORIENTED_EDGE ( 'NONE', *, *, #39357, .F. ) ;
#186926=CARTESIAN_POINT ( 'NONE',  ( 19.29714446218642721, -35.03787052511701461, -7.260590851364162823 ) ) ;
#187072=CARTESIAN_POINT ( 'NONE',  ( -3.573655867282028392E-15, 2.428612866367529932E-14, 1.984260520772446048E-44 ) ) ;
#187152=ADVANCED_FACE ( 'NONE', ( #43764 ), #153696, .T. ) ;
#187216=CARTESIAN_POINT ( 'NONE',  ( -4.911121358187451425E-30, -78.67194367458512261, -13.00000000000000000 ) ) ;
#187511=DIRECTION ( 'NONE',  ( -1.000000000000000000, 0.000000000000000000, 0.000000000000000000 ) ) ;
#187578=LINE ( 'NONE', #94534, #108855 ) ;
#187587=DIRECTION ( 'NONE',  ( 0.000000000000000000, 0.000000000000000000, 1.000000000000000000 ) ) ;
#187784=CARTESIAN_POINT ( 'NONE',  ( -3.573655867282013404E-15, -180.0000000000000000, -15.00000000000000000 ) ) ;
#187808=CARTESIAN_POINT ( 'NONE',  ( -11.30153831258470731, -180.0000000000000568, -4.999999999999999112 ) ) ;
#187911=DIRECTION ( 'NONE',  ( -1.000000000000000000, 5.392603844284257652E-33, 0.000000000000000000 ) ) ;
#188027=CARTESIAN_POINT ( 'NONE',  ( 69.65682714487590488, -71.74905178543389184, -15.00000000000000000 ) ) ;
#188030=CARTESIAN_POINT ( 'NONE',  ( -27.86273085795037474, -28.69962071417356242, -4.999999999999999112 ) ) ;
#188073=ORIENTED_EDGE ( 'NONE', *, *, #178304, .F. ) ;
#188244=PLANE ( 'NONE',  #164368 ) ;
#188252=DIRECTION ( 'NONE',  ( 0.000000000000000000, 0.000000000000000000, 1.000000000000000000 ) ) ;
#188443=VERTEX_POINT ( 'NONE', #22118 ) ;
#188447=VERTEX_POINT ( 'NONE', #131284 ) ;
#188802=ORIENTED_EDGE ( 'NONE', *, *, #164988, .T. ) ;
#188902=TOROIDAL_SURFACE ( 'NONE', #95210, 206.0437394197456342, 10.00000000000000000 ) ;
#188905=CARTESIAN_POINT ( 'NONE',  ( 19.92827645216230437, -34.68249012782280261, -5.691795689800142277 ) ) ;
#188985=VECTOR ( 'NONE', #64859, 1000.000000000000000 ) ;
#189313=EDGE_CURVE ( 'NONE', #38864, #27838, #8368, .T. ) ;
#189502=ORIENTED_EDGE ( 'NONE', *, *, #46506, .T. ) ;
#189513=ADVANCED_BREP_SHAPE_REPRESENTATION ( '', ( #7058, #82054 ), #50057 ) ;
#189649=CIRCLE ( 'NONE', #170294, 2.649999999999999911 ) ;
#189718=CARTESIAN_POINT ( 'NONE',  ( 193.3062444957835453, -155.7167183371837496, 0.000000000000000000 ) ) ;
#189784=AXIS2_PLACEMENT_3D ( 'NONE', #158181, #23668, #147008 ) ;
#189948=CIRCLE ( 'NONE', #60759, 1.000000000000000888 ) ;
#190067=DIRECTION ( 'NONE',  ( 5.204170427930421283E-16, 7.149051953565419487E-31, -1.000000000000000000 ) ) ;
#190116=CYLINDRICAL_SURFACE ( 'NONE', #151814, 10.00000000000000000 ) ;
#190304=ORIENTED_EDGE ( 'NONE', *, *, #59958, .T. ) ;
#190441=ORIENTED_EDGE ( 'NONE', *, *, #198923, .T. ) ;
#190486=CARTESIAN_POINT ( 'NONE',  ( -12.23824476834559150, -38.08322923102583957, -12.22663129986431052 ) ) ;
#190541=CARTESIAN_POINT ( 'NONE',  ( -5.000000000000000888, -130.0000000000000000, -13.99999999999999822 ) ) ;
#190601=AXIS2_PLACEMENT_3D ( 'NONE', #4433, #139973, #18645 ) ;
#190895=DIRECTION ( 'NONE',  ( 0.000000000000000000, 0.000000000000000000, 1.000000000000000000 ) ) ;
#191008=CARTESIAN_POINT ( 'NONE',  ( 2.539210307071009592E-15, -74.04165629597449083, -14.99410988461187699 ) ) ;
#191029=CARTESIAN_POINT ( 'NONE',  ( 5.000000000000000888, -140.0000000000000000, -13.00000000000000000 ) ) ;
#191034=FILL_AREA_STYLE_COLOUR ( '', #159726 ) ;
#191110=VECTOR ( 'NONE', #171917, 1000.000000000000000 ) ;
#191369=DIRECTION ( 'NONE',  ( -1.000000000000000000, 0.000000000000000000, 0.000000000000000000 ) ) ;
#191582=AXIS2_PLACEMENT_3D ( 'NONE', #4543, #130897, #83386 ) ;
#191766=CARTESIAN_POINT ( 'NONE',  ( 5.000000000000000888, -130.0000000000000000, -13.99999999999999822 ) ) ;
#191773=FACE_OUTER_BOUND ( 'NONE', #128919, .T. ) ;
#191777=DIRECTION ( 'NONE',  ( -1.000000000000000000, 0.000000000000000000, 0.000000000000000000 ) ) ;
#191780=CIRCLE ( 'NONE', #104637, 10.00000000000000000 ) ;
#191850=DIRECTION ( 'NONE',  ( -4.336808689942017120E-17, -1.000000000000000000, 0.000000000000000000 ) ) ;
#191917=CIRCLE ( 'NONE', #175909, 8.000000000000000000 ) ;
#192038=VERTEX_POINT ( 'NONE', #138661 ) ;
#192093=AXIS2_PLACEMENT_3D ( 'NONE', #43775, #107406, #92237 ) ;
#192669=EDGE_LOOP ( 'NONE', ( #81317, #22697, #59702, #59498, #111591 ) ) ;
#192727=AXIS2_PLACEMENT_3D ( 'NONE', #190541, #6497, #173389 ) ;
#192802=ORIENTED_EDGE ( 'NONE', *, *, #48191, .T. ) ;
#192870=CIRCLE ( 'NONE', #25032, 8.000000000000000000 ) ;
#193014=DIRECTION ( 'NONE',  ( -1.000000000000000000, 0.000000000000000000, 0.000000000000000000 ) ) ;
#193308=DIRECTION ( 'NONE',  ( 1.000000000000000000, 0.000000000000000000, 0.000000000000000000 ) ) ;
#193309=EDGE_LOOP ( 'NONE', ( #70675, #47948, #138259, #171474, #194481 ) ) ;
#193366=CARTESIAN_POINT ( 'NONE',  ( 27.86273085795037119, -28.69962071417355531, 0.000000000000000000 ) ) ;
#193385=DIRECTION ( 'NONE',  ( 1.000000000000000000, 0.000000000000000000, 0.000000000000000000 ) ) ;
#193468=CARTESIAN_POINT ( 'NONE',  ( -2.973862142520655727, -93.04182470242767522, -4.999999999999999112 ) ) ;
#193478=VERTEX_POINT ( 'NONE', #67615 ) ;
#193511=DIRECTION ( 'NONE',  ( -0.000000000000000000, -0.000000000000000000, -1.000000000000000000 ) ) ;
#193517=VERTEX_POINT ( 'NONE', #158630 ) ;
#193705=DIRECTION ( 'NONE',  ( 0.000000000000000000, 0.000000000000000000, -1.000000000000000000 ) ) ;
#193790=B_SPLINE_CURVE_WITH_KNOTS ( 'NONE', 3,
 ( #113156, #191008, #128323, #84805, #68649, #115163, #146484 ),
 .UNSPECIFIED., .F., .F.,
 ( 4, 3, 4 ),
 ( 0.006877813788783073562, 0.01375562809188920002, 0.01380070845639014970 ),
 .UNSPECIFIED. ) ;
#193969=FACE_BOUND ( 'NONE', #97688, .T. ) ;
#194481=ORIENTED_EDGE ( 'NONE', *, *, #955, .F. ) ;
#194519=ORIENTED_EDGE ( 'NONE', *, *, #100961, .F. ) ;
#194585=DIRECTION ( 'NONE',  ( -1.000000000000000000, 0.000000000000000000, 0.000000000000000000 ) ) ;
#194813=ORIENTED_EDGE ( 'NONE', *, *, #163970, .T. ) ;
#195043=CARTESIAN_POINT ( 'NONE',  ( -27.86473085795038429, -130.0000000000000000, -13.99999999999999822 ) ) ;
#195156=VECTOR ( 'NONE', #112941, 1000.000000000000000 ) ;
#195359=AXIS2_PLACEMENT_3D ( 'NONE', #89122, #73972, #91083 ) ;
#195401=CIRCLE ( 'NONE', #11382, 2.649999999999999911 ) ;
#195451=AXIS2_PLACEMENT_3D ( 'NONE', #67389, #173596, #35065 ) ;
#195493=TOROIDAL_SURFACE ( 'NONE', #72809, 69.99999999999998579, 8.000000000000000000 ) ;
#195692=ORIENTED_EDGE ( 'NONE', *, *, #85978, .T. ) ;
#195786=AXIS2_PLACEMENT_3D ( 'NONE', #50985, #81293, #142977 ) ;
#195929=AXIS2_PLACEMENT_3D ( 'NONE', #30615, #1246, #60938 ) ;
#195984=ORIENTED_EDGE ( 'NONE', *, *, #66709, .F. ) ;
#196229=CIRCLE ( 'NONE', #83140, 69.99999999999998579 ) ;
#196650=EDGE_CURVE ( 'NONE', #127511, #54470, #158355, .T. ) ;
#197076=CARTESIAN_POINT ( 'NONE',  ( -6.856101608890819192E-16, -64.86648100006283357, -12.99999901186700946 ) ) ;
#197144=ORIENTED_EDGE ( 'NONE', *, *, #78587, .F. ) ;
#197193=VERTEX_POINT ( 'NONE', #153933 ) ;
#197311=DIRECTION ( 'NONE',  ( -1.000000000000000000, 0.000000000000000000, 0.000000000000000000 ) ) ;
#197466=FACE_OUTER_BOUND ( 'NONE', #106289, .T. ) ;
#197544=PLANE ( 'NONE',  #153039 ) ;
#197698=DIRECTION ( 'NONE',  ( -1.000000000000000000, 0.000000000000000000, 0.000000000000000000 ) ) ;
#197850=DIRECTION ( 'NONE',  ( 4.336808689942017120E-17, 1.000000000000000000, 0.000000000000000000 ) ) ;
#197949=VERTEX_POINT ( 'NONE', #119403 ) ;
#197996=CARTESIAN_POINT ( 'NONE',  ( -193.3062444957834884, -155.7167183371838064, -4.999999999999999112 ) ) ;
#198064=DIRECTION ( 'NONE',  ( 0.000000000000000000, 0.000000000000000000, -1.000000000000000000 ) ) ;
#198276=DIRECTION ( 'NONE',  ( 0.000000000000000000, 0.000000000000000000, -1.000000000000000000 ) ) ;
#198310=VECTOR ( 'NONE', #116028, 1000.000000000000000 ) ;
#198450=PLANE ( 'NONE',  #192093 ) ;
#198460=CARTESIAN_POINT ( 'NONE',  ( -19.97888994334923751, -34.65319547504295628, -4.999999999999999112 ) ) ;
#198479=DIRECTION ( 'NONE',  ( -1.000000000000000000, 0.000000000000000000, 0.000000000000000000 ) ) ;
#198492=EDGE_LOOP ( 'NONE', ( #130978, #60108, #170649, #28640 ) ) ;
#198527=ADVANCED_FACE ( 'NONE', ( #122355 ), #45527, .F. ) ;
#198529=CARTESIAN_POINT ( 'NONE',  ( -11.30153831258471442, -180.0000000000000000, -13.00000000000000000 ) ) ;
#198768=DIRECTION ( 'NONE',  ( 0.000000000000000000, 0.000000000000000000, -1.000000000000000000 ) ) ;
#198923=EDGE_CURVE ( 'NONE', #166994, #197193, #126812, .T. ) ;
#198974=FACE_OUTER_BOUND ( 'NONE', #85422, .T. ) ;
#199019=DIRECTION ( 'NONE',  ( -1.000000000000000000, 0.000000000000000000, 0.000000000000000000 ) ) ;
#199031=CIRCLE ( 'NONE', #160334, 8.000000000000000000 ) ;
#199051=CARTESIAN_POINT ( 'NONE',  ( -4.814824860968089633E-30, -78.67194367458512261, -15.00000000000000000 ) ) ;
#199177=VECTOR ( 'NONE', #184104, 1000.000000000000000 ) ;
#199198=DIRECTION ( 'NONE',  ( 0.000000000000000000, 0.000000000000000000, 1.000000000000000000 ) ) ;
#199319=ORIENTED_EDGE ( 'NONE', *, *, #106368, .F. ) ;
#199403=ORIENTED_EDGE ( 'NONE', *, *, #68983, .T. ) ;
#199432=LINE ( 'NONE', #10449, #157478 ) ;
#199477=CIRCLE ( 'NONE', #170464, 206.0437394197456342 ) ;
#199556=DIRECTION ( 'NONE',  ( 0.000000000000000000, 0.000000000000000000, 1.000000000000000000 ) ) ;
#199602=AXIS2_PLACEMENT_3D ( 'NONE', #55659, #39488, #54657 ) ;
#199827=EDGE_CURVE ( 'NONE', #40357, #142969, #191780, .T. ) ;
#199907=CYLINDRICAL_SURFACE ( 'NONE', #20852, 2.649999999999999911 ) ;
#200108=ORIENTED_EDGE ( 'NONE', *, *, #139548, .F. ) ;
ENDSEC;
END-ISO-10303-21;
